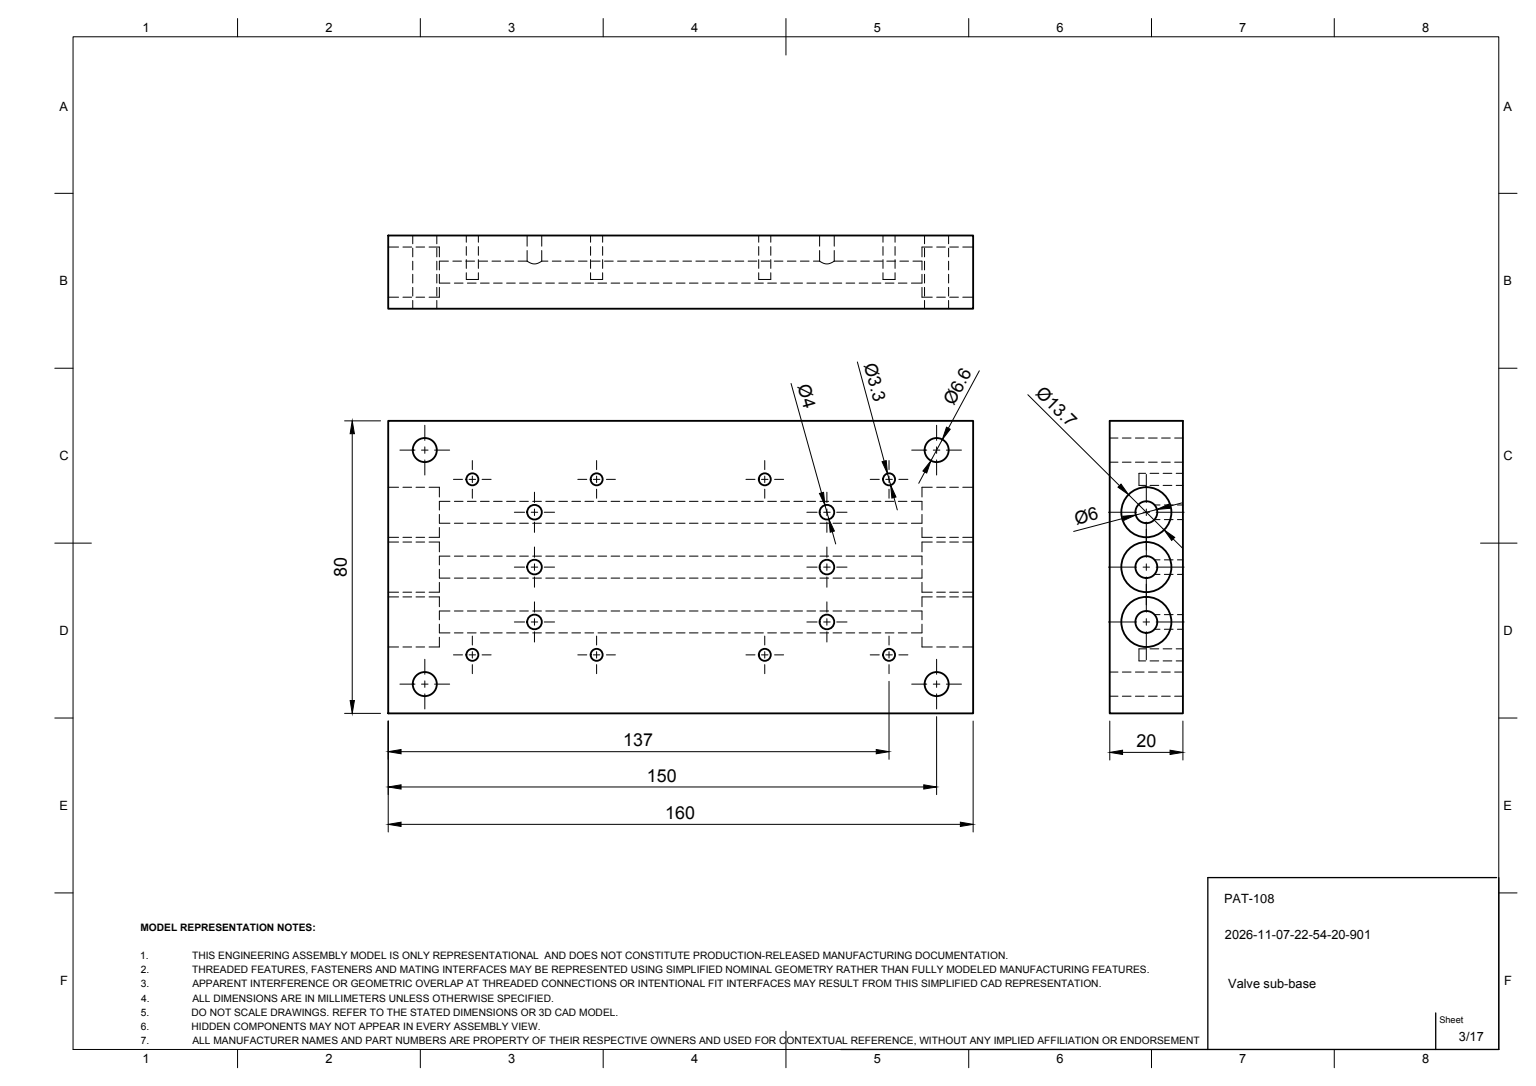
ISO-10303-21;
HEADER;
/* Generated by software containing ST-Developer
 * from STEP Tools, Inc. (www.steptools.com) 
 */

FILE_DESCRIPTION(
/* description */ ('Sub-base valve envelopes and connections'),
/* implementation_level */ '2;1');

FILE_NAME(
/* name */ 'Valve sub-base.step',
/* time_stamp */ '2026-10-29T15:55:44-07:00',
/* author */ (''),
/* organization */ (''),
/* preprocessor_version */ 'ST-DEVELOPER v20.2',
/* originating_system */ 'Autodesk Translation Framework v15.17.0.0',
/* authorisation */ '');

FILE_SCHEMA (('AUTOMOTIVE_DESIGN { 1 0 10303 214 3 1 1 }'));
ENDSEC;

DATA;
#10=MECHANICAL_DESIGN_GEOMETRIC_PRESENTATION_REPRESENTATION('',(#119),#6113);
#95=SHAPE_REPRESENTATION_RELATIONSHIP('SRR','None',#6168,#107);
#107=ADVANCED_BREP_SHAPE_REPRESENTATION('',(#131),#6099);
#119=STYLED_ITEM('',(#6294),#131);
#131=MANIFOLD_SOLID_BREP('Body1',#3358);
#142=FACE_BOUND('',#613,.T.);
#143=FACE_BOUND('',#616,.T.);
#144=FACE_BOUND('',#619,.T.);
#145=FACE_BOUND('',#622,.T.);
#146=FACE_BOUND('',#625,.T.);
#147=FACE_BOUND('',#628,.T.);
#148=FACE_BOUND('',#634,.T.);
#149=FACE_BOUND('',#635,.T.);
#150=FACE_BOUND('',#636,.T.);
#151=FACE_BOUND('',#639,.T.);
#152=FACE_BOUND('',#640,.T.);
#153=FACE_BOUND('',#641,.T.);
#154=FACE_BOUND('',#643,.T.);
#155=FACE_BOUND('',#644,.T.);
#156=FACE_BOUND('',#645,.T.);
#157=FACE_BOUND('',#646,.T.);
#158=FACE_BOUND('',#647,.T.);
#159=FACE_BOUND('',#648,.T.);
#160=FACE_BOUND('',#649,.T.);
#161=FACE_BOUND('',#650,.T.);
#162=FACE_BOUND('',#651,.T.);
#163=FACE_BOUND('',#652,.T.);
#164=FACE_BOUND('',#653,.T.);
#165=FACE_BOUND('',#654,.T.);
#166=FACE_BOUND('',#655,.T.);
#167=FACE_BOUND('',#656,.T.);
#168=FACE_BOUND('',#657,.T.);
#169=FACE_BOUND('',#658,.T.);
#170=FACE_BOUND('',#659,.T.);
#171=FACE_BOUND('',#660,.T.);
#172=FACE_BOUND('',#662,.T.);
#173=FACE_BOUND('',#663,.T.);
#174=FACE_BOUND('',#664,.T.);
#175=FACE_BOUND('',#665,.T.);
#259=B_SPLINE_CURVE_WITH_KNOTS('',3,(#4974,#4975,#4976,#4977,#4978,#4979,
#4980,#4981,#4982,#4983),.UNSPECIFIED.,.F.,.F.,(4,2,2,2,4),(0.,0.0789054703932594,
0.157810940786519,0.235848341776527,0.313885742766534),.UNSPECIFIED.);
#260=B_SPLINE_CURVE_WITH_KNOTS('',3,(#4985,#4986,#4987,#4988,#4989,#4990,
#4991,#4992,#4993,#4994),.UNSPECIFIED.,.F.,.F.,(4,2,2,2,4),(0.941657228299604,
1.01969462928961,1.09773203027962,1.17663750067288,1.25554297106614),
 .UNSPECIFIED.);
#261=B_SPLINE_CURVE_WITH_KNOTS('',3,(#4998,#4999,#5000,#5001,#5002,#5003,
#5004,#5005,#5006,#5007,#5008,#5009,#5010,#5011,#5012,#5013,#5014,#5015),
 .UNSPECIFIED.,.F.,.F.,(4,2,2,2,2,2,2,2,4),(0.313885742766534,0.391923143756543,
0.469960544746551,0.54886601513981,0.627771485533069,0.706676955926329,
0.785582426319588,0.863619827309596,0.941657228299604),.UNSPECIFIED.);
#262=B_SPLINE_CURVE_WITH_KNOTS('',3,(#5019,#5020,#5021,#5022,#5023,#5024,
#5025,#5026,#5027,#5028),.UNSPECIFIED.,.F.,.F.,(4,2,2,2,4),(0.,0.0789054703932594,
0.157810940786519,0.235848341776527,0.313885742766535),.UNSPECIFIED.);
#263=B_SPLINE_CURVE_WITH_KNOTS('',3,(#5030,#5031,#5032,#5033,#5034,#5035,
#5036,#5037,#5038,#5039),.UNSPECIFIED.,.F.,.F.,(4,2,2,2,4),(0.941657228299605,
1.01969462928961,1.09773203027962,1.17663750067288,1.25554297106614),
 .UNSPECIFIED.);
#264=B_SPLINE_CURVE_WITH_KNOTS('',3,(#5043,#5044,#5045,#5046,#5047,#5048,
#5049,#5050,#5051,#5052,#5053,#5054,#5055,#5056,#5057,#5058,#5059,#5060),
 .UNSPECIFIED.,.F.,.F.,(4,2,2,2,2,2,2,2,4),(0.313885742766535,0.391923143756543,
0.469960544746551,0.54886601513981,0.627771485533069,0.706676955926329,
0.785582426319588,0.863619827309597,0.941657228299605),.UNSPECIFIED.);
#265=B_SPLINE_CURVE_WITH_KNOTS('',3,(#5064,#5065,#5066,#5067,#5068,#5069,
#5070,#5071,#5072,#5073),.UNSPECIFIED.,.F.,.F.,(4,2,2,2,4),(0.,0.0789054703932594,
0.157810940786519,0.235848341776527,0.313885742766534),.UNSPECIFIED.);
#266=B_SPLINE_CURVE_WITH_KNOTS('',3,(#5075,#5076,#5077,#5078,#5079,#5080,
#5081,#5082,#5083,#5084),.UNSPECIFIED.,.F.,.F.,(4,2,2,2,4),(0.941657228299604,
1.01969462928961,1.09773203027962,1.17663750067288,1.25554297106614),
 .UNSPECIFIED.);
#267=B_SPLINE_CURVE_WITH_KNOTS('',3,(#5088,#5089,#5090,#5091,#5092,#5093,
#5094,#5095,#5096,#5097,#5098,#5099,#5100,#5101,#5102,#5103,#5104,#5105),
 .UNSPECIFIED.,.F.,.F.,(4,2,2,2,2,2,2,2,4),(0.313885742766534,0.391923143756543,
0.469960544746551,0.54886601513981,0.627771485533069,0.706676955926329,
0.785582426319588,0.863619827309596,0.941657228299604),.UNSPECIFIED.);
#268=B_SPLINE_CURVE_WITH_KNOTS('',3,(#5137,#5138,#5139,#5140,#5141,#5142,
#5143,#5144,#5145,#5146),.UNSPECIFIED.,.F.,.F.,(4,2,2,2,4),(0.,0.0789054703932594,
0.157810940786519,0.235848341776527,0.313885742766535),.UNSPECIFIED.);
#269=B_SPLINE_CURVE_WITH_KNOTS('',3,(#5148,#5149,#5150,#5151,#5152,#5153,
#5154,#5155,#5156,#5157),.UNSPECIFIED.,.F.,.F.,(4,2,2,2,4),(0.941657228299605,
1.01969462928961,1.09773203027962,1.17663750067288,1.25554297106614),
 .UNSPECIFIED.);
#270=B_SPLINE_CURVE_WITH_KNOTS('',3,(#5161,#5162,#5163,#5164,#5165,#5166,
#5167,#5168,#5169,#5170,#5171,#5172,#5173,#5174,#5175,#5176,#5177,#5178),
 .UNSPECIFIED.,.F.,.F.,(4,2,2,2,2,2,2,2,4),(0.313885742766535,0.391923143756543,
0.469960544746551,0.54886601513981,0.62777148553307,0.706676955926329,0.785582426319589,
0.863619827309597,0.941657228299605),.UNSPECIFIED.);
#271=B_SPLINE_CURVE_WITH_KNOTS('',3,(#5182,#5183,#5184,#5185,#5186,#5187,
#5188,#5189,#5190,#5191),.UNSPECIFIED.,.F.,.F.,(4,2,2,2,4),(0.,0.0789054703932594,
0.157810940786519,0.235848341776527,0.313885742766535),.UNSPECIFIED.);
#272=B_SPLINE_CURVE_WITH_KNOTS('',3,(#5193,#5194,#5195,#5196,#5197,#5198,
#5199,#5200,#5201,#5202),.UNSPECIFIED.,.F.,.F.,(4,2,2,2,4),(0.941657228299605,
1.01969462928961,1.09773203027962,1.17663750067288,1.25554297106614),
 .UNSPECIFIED.);
#273=B_SPLINE_CURVE_WITH_KNOTS('',3,(#5206,#5207,#5208,#5209,#5210,#5211,
#5212,#5213,#5214,#5215,#5216,#5217,#5218,#5219,#5220,#5221,#5222,#5223),
 .UNSPECIFIED.,.F.,.F.,(4,2,2,2,2,2,2,2,4),(0.313885742766535,0.391923143756543,
0.469960544746551,0.548866015139811,0.62777148553307,0.706676955926329,
0.785582426319589,0.863619827309597,0.941657228299605),.UNSPECIFIED.);
#274=B_SPLINE_CURVE_WITH_KNOTS('',3,(#5227,#5228,#5229,#5230,#5231,#5232,
#5233,#5234,#5235,#5236),.UNSPECIFIED.,.F.,.F.,(4,2,2,2,4),(0.,0.0789054703932594,
0.157810940786519,0.235848341776527,0.313885742766535),.UNSPECIFIED.);
#275=B_SPLINE_CURVE_WITH_KNOTS('',3,(#5238,#5239,#5240,#5241,#5242,#5243,
#5244,#5245,#5246,#5247),.UNSPECIFIED.,.F.,.F.,(4,2,2,2,4),(0.941657228299605,
1.01969462928961,1.09773203027962,1.17663750067288,1.25554297106614),
 .UNSPECIFIED.);
#276=B_SPLINE_CURVE_WITH_KNOTS('',3,(#5251,#5252,#5253,#5254,#5255,#5256,
#5257,#5258,#5259,#5260,#5261,#5262,#5263,#5264,#5265,#5266,#5267,#5268),
 .UNSPECIFIED.,.F.,.F.,(4,2,2,2,2,2,2,2,4),(0.313885742766535,0.391923143756543,
0.469960544746551,0.54886601513981,0.62777148553307,0.706676955926329,0.785582426319589,
0.863619827309597,0.941657228299605),.UNSPECIFIED.);
#277=PLANE('',#3509);
#278=PLANE('',#3513);
#279=PLANE('',#3517);
#280=PLANE('',#3521);
#281=PLANE('',#3531);
#282=PLANE('',#3535);
#283=PLANE('',#3539);
#284=PLANE('',#3543);
#285=PLANE('',#3565);
#286=PLANE('',#3570);
#287=PLANE('',#3575);
#288=PLANE('',#3580);
#289=PLANE('',#3585);
#290=PLANE('',#3590);
#291=PLANE('',#3595);
#292=PLANE('',#3596);
#293=PLANE('',#3597);
#294=PLANE('',#3598);
#295=PLANE('',#3599);
#296=PLANE('',#3600);
#386=FACE_OUTER_BOUND('',#585,.T.);
#387=FACE_OUTER_BOUND('',#586,.T.);
#388=FACE_OUTER_BOUND('',#587,.T.);
#389=FACE_OUTER_BOUND('',#588,.T.);
#390=FACE_OUTER_BOUND('',#589,.T.);
#391=FACE_OUTER_BOUND('',#590,.T.);
#392=FACE_OUTER_BOUND('',#591,.T.);
#393=FACE_OUTER_BOUND('',#592,.T.);
#394=FACE_OUTER_BOUND('',#593,.T.);
#395=FACE_OUTER_BOUND('',#594,.T.);
#396=FACE_OUTER_BOUND('',#595,.T.);
#397=FACE_OUTER_BOUND('',#596,.T.);
#398=FACE_OUTER_BOUND('',#597,.T.);
#399=FACE_OUTER_BOUND('',#598,.T.);
#400=FACE_OUTER_BOUND('',#599,.T.);
#401=FACE_OUTER_BOUND('',#600,.T.);
#402=FACE_OUTER_BOUND('',#601,.T.);
#403=FACE_OUTER_BOUND('',#602,.T.);
#404=FACE_OUTER_BOUND('',#603,.T.);
#405=FACE_OUTER_BOUND('',#604,.T.);
#406=FACE_OUTER_BOUND('',#605,.T.);
#407=FACE_OUTER_BOUND('',#606,.T.);
#408=FACE_OUTER_BOUND('',#607,.T.);
#409=FACE_OUTER_BOUND('',#608,.T.);
#410=FACE_OUTER_BOUND('',#609,.T.);
#411=FACE_OUTER_BOUND('',#610,.T.);
#412=FACE_OUTER_BOUND('',#611,.T.);
#413=FACE_OUTER_BOUND('',#612,.T.);
#414=FACE_OUTER_BOUND('',#614,.T.);
#415=FACE_OUTER_BOUND('',#615,.T.);
#416=FACE_OUTER_BOUND('',#617,.T.);
#417=FACE_OUTER_BOUND('',#618,.T.);
#418=FACE_OUTER_BOUND('',#620,.T.);
#419=FACE_OUTER_BOUND('',#621,.T.);
#420=FACE_OUTER_BOUND('',#623,.T.);
#421=FACE_OUTER_BOUND('',#624,.T.);
#422=FACE_OUTER_BOUND('',#626,.T.);
#423=FACE_OUTER_BOUND('',#627,.T.);
#424=FACE_OUTER_BOUND('',#629,.T.);
#425=FACE_OUTER_BOUND('',#630,.T.);
#426=FACE_OUTER_BOUND('',#631,.T.);
#427=FACE_OUTER_BOUND('',#632,.T.);
#428=FACE_OUTER_BOUND('',#633,.T.);
#429=FACE_OUTER_BOUND('',#637,.T.);
#430=FACE_OUTER_BOUND('',#638,.T.);
#431=FACE_OUTER_BOUND('',#642,.T.);
#432=FACE_OUTER_BOUND('',#661,.T.);
#585=EDGE_LOOP('',(#2235,#2236,#2237,#2238));
#586=EDGE_LOOP('',(#2239));
#587=EDGE_LOOP('',(#2240,#2241,#2242,#2243));
#588=EDGE_LOOP('',(#2244));
#589=EDGE_LOOP('',(#2245,#2246,#2247,#2248));
#590=EDGE_LOOP('',(#2249));
#591=EDGE_LOOP('',(#2250,#2251,#2252,#2253));
#592=EDGE_LOOP('',(#2254));
#593=EDGE_LOOP('',(#2255,#2256,#2257,#2258,#2259,#2260));
#594=EDGE_LOOP('',(#2261,#2262,#2263,#2264,#2265,#2266));
#595=EDGE_LOOP('',(#2267,#2268,#2269,#2270,#2271,#2272));
#596=EDGE_LOOP('',(#2273,#2274,#2275,#2276));
#597=EDGE_LOOP('',(#2277));
#598=EDGE_LOOP('',(#2278,#2279,#2280,#2281));
#599=EDGE_LOOP('',(#2282));
#600=EDGE_LOOP('',(#2283,#2284,#2285,#2286));
#601=EDGE_LOOP('',(#2287));
#602=EDGE_LOOP('',(#2288,#2289,#2290,#2291));
#603=EDGE_LOOP('',(#2292));
#604=EDGE_LOOP('',(#2293,#2294,#2295,#2296,#2297,#2298));
#605=EDGE_LOOP('',(#2299,#2300,#2301,#2302,#2303,#2304));
#606=EDGE_LOOP('',(#2305,#2306,#2307,#2308,#2309,#2310));
#607=EDGE_LOOP('',(#2311,#2312,#2313,#2314));
#608=EDGE_LOOP('',(#2315,#2316,#2317,#2318));
#609=EDGE_LOOP('',(#2319,#2320,#2321,#2322));
#610=EDGE_LOOP('',(#2323,#2324,#2325,#2326));
#611=EDGE_LOOP('',(#2327,#2328,#2329,#2330));
#612=EDGE_LOOP('',(#2331));
#613=EDGE_LOOP('',(#2332));
#614=EDGE_LOOP('',(#2333,#2334,#2335,#2336));
#615=EDGE_LOOP('',(#2337));
#616=EDGE_LOOP('',(#2338));
#617=EDGE_LOOP('',(#2339,#2340,#2341,#2342));
#618=EDGE_LOOP('',(#2343));
#619=EDGE_LOOP('',(#2344));
#620=EDGE_LOOP('',(#2345,#2346,#2347,#2348));
#621=EDGE_LOOP('',(#2349));
#622=EDGE_LOOP('',(#2350));
#623=EDGE_LOOP('',(#2351,#2352,#2353,#2354));
#624=EDGE_LOOP('',(#2355));
#625=EDGE_LOOP('',(#2356));
#626=EDGE_LOOP('',(#2357,#2358,#2359,#2360));
#627=EDGE_LOOP('',(#2361));
#628=EDGE_LOOP('',(#2362));
#629=EDGE_LOOP('',(#2363,#2364,#2365,#2366,#2367,#2368,#2369,#2370,#2371,
#2372,#2373,#2374,#2375,#2376));
#630=EDGE_LOOP('',(#2377,#2378,#2379,#2380,#2381,#2382,#2383,#2384,#2385,
#2386,#2387,#2388,#2389,#2390));
#631=EDGE_LOOP('',(#2391,#2392,#2393,#2394,#2395,#2396,#2397,#2398,#2399,
#2400,#2401,#2402,#2403,#2404));
#632=EDGE_LOOP('',(#2405,#2406,#2407,#2408));
#633=EDGE_LOOP('',(#2409,#2410,#2411,#2412));
#634=EDGE_LOOP('',(#2413));
#635=EDGE_LOOP('',(#2414));
#636=EDGE_LOOP('',(#2415));
#637=EDGE_LOOP('',(#2416,#2417,#2418,#2419));
#638=EDGE_LOOP('',(#2420,#2421,#2422,#2423));
#639=EDGE_LOOP('',(#2424));
#640=EDGE_LOOP('',(#2425));
#641=EDGE_LOOP('',(#2426));
#642=EDGE_LOOP('',(#2427,#2428,#2429,#2430));
#643=EDGE_LOOP('',(#2431));
#644=EDGE_LOOP('',(#2432));
#645=EDGE_LOOP('',(#2433));
#646=EDGE_LOOP('',(#2434));
#647=EDGE_LOOP('',(#2435));
#648=EDGE_LOOP('',(#2436));
#649=EDGE_LOOP('',(#2437));
#650=EDGE_LOOP('',(#2438));
#651=EDGE_LOOP('',(#2439));
#652=EDGE_LOOP('',(#2440));
#653=EDGE_LOOP('',(#2441));
#654=EDGE_LOOP('',(#2442));
#655=EDGE_LOOP('',(#2443));
#656=EDGE_LOOP('',(#2444));
#657=EDGE_LOOP('',(#2445));
#658=EDGE_LOOP('',(#2446));
#659=EDGE_LOOP('',(#2447));
#660=EDGE_LOOP('',(#2448));
#661=EDGE_LOOP('',(#2449,#2450,#2451,#2452));
#662=EDGE_LOOP('',(#2453));
#663=EDGE_LOOP('',(#2454));
#664=EDGE_LOOP('',(#2455));
#665=EDGE_LOOP('',(#2456));
#901=LINE('',#4947,#1135);
#902=LINE('',#4954,#1136);
#903=LINE('',#4961,#1137);
#904=LINE('',#4968,#1138);
#905=LINE('',#4996,#1139);
#906=LINE('',#5041,#1140);
#907=LINE('',#5086,#1141);
#908=LINE('',#5110,#1142);
#909=LINE('',#5117,#1143);
#910=LINE('',#5124,#1144);
#911=LINE('',#5131,#1145);
#912=LINE('',#5159,#1146);
#913=LINE('',#5204,#1147);
#914=LINE('',#5249,#1148);
#915=LINE('',#5273,#1149);
#916=LINE('',#5279,#1150);
#917=LINE('',#5285,#1151);
#918=LINE('',#5291,#1152);
#919=LINE('',#5297,#1153);
#920=LINE('',#5306,#1154);
#921=LINE('',#5315,#1155);
#922=LINE('',#5324,#1156);
#923=LINE('',#5333,#1157);
#924=LINE('',#5342,#1158);
#925=LINE('',#5348,#1159);
#926=LINE('',#5349,#1160);
#927=LINE('',#5350,#1161);
#928=LINE('',#5352,#1162);
#929=LINE('',#5353,#1163);
#930=LINE('',#5354,#1164);
#931=LINE('',#5356,#1165);
#932=LINE('',#5357,#1166);
#933=LINE('',#5358,#1167);
#934=LINE('',#5362,#1168);
#935=LINE('',#5364,#1169);
#936=LINE('',#5366,#1170);
#937=LINE('',#5367,#1171);
#938=LINE('',#5370,#1172);
#939=LINE('',#5372,#1173);
#940=LINE('',#5373,#1174);
#941=LINE('',#5376,#1175);
#942=LINE('',#5378,#1176);
#943=LINE('',#5379,#1177);
#944=LINE('',#5381,#1178);
#945=LINE('',#5382,#1179);
#1135=VECTOR('',#3913,0.165);
#1136=VECTOR('',#3922,0.165);
#1137=VECTOR('',#3931,0.165);
#1138=VECTOR('',#3940,0.165);
#1139=VECTOR('',#3947,0.2);
#1140=VECTOR('',#3952,0.2);
#1141=VECTOR('',#3957,0.2);
#1142=VECTOR('',#3964,0.165);
#1143=VECTOR('',#3973,0.165);
#1144=VECTOR('',#3982,0.165);
#1145=VECTOR('',#3991,0.165);
#1146=VECTOR('',#3998,0.2);
#1147=VECTOR('',#4003,0.2);
#1148=VECTOR('',#4008,0.2);
#1149=VECTOR('',#4015,0.33);
#1150=VECTOR('',#4022,0.33);
#1151=VECTOR('',#4029,0.33);
#1152=VECTOR('',#4036,0.33);
#1153=VECTOR('',#4043,0.685);
#1154=VECTOR('',#4054,0.685);
#1155=VECTOR('',#4065,0.685);
#1156=VECTOR('',#4076,0.685);
#1157=VECTOR('',#4087,0.685);
#1158=VECTOR('',#4098,0.685);
#1159=VECTOR('',#4107,0.3);
#1160=VECTOR('',#4108,0.3);
#1161=VECTOR('',#4109,0.3);
#1162=VECTOR('',#4112,0.3);
#1163=VECTOR('',#4113,0.3);
#1164=VECTOR('',#4114,0.3);
#1165=VECTOR('',#4117,0.3);
#1166=VECTOR('',#4118,0.3);
#1167=VECTOR('',#4119,0.3);
#1168=VECTOR('',#4122,1.);
#1169=VECTOR('',#4123,1.);
#1170=VECTOR('',#4124,1.);
#1171=VECTOR('',#4125,1.);
#1172=VECTOR('',#4128,1.);
#1173=VECTOR('',#4129,1.);
#1174=VECTOR('',#4130,1.);
#1175=VECTOR('',#4133,1.);
#1176=VECTOR('',#4134,1.);
#1177=VECTOR('',#4135,1.);
#1178=VECTOR('',#4138,1.);
#1179=VECTOR('',#4139,1.);
#1369=CIRCLE('',#3507,0.165);
#1370=CIRCLE('',#3508,0.165);
#1371=CIRCLE('',#3511,0.165);
#1372=CIRCLE('',#3512,0.165);
#1373=CIRCLE('',#3515,0.165);
#1374=CIRCLE('',#3516,0.165);
#1375=CIRCLE('',#3519,0.165);
#1376=CIRCLE('',#3520,0.165);
#1377=CIRCLE('',#3523,0.2);
#1378=CIRCLE('',#3525,0.2);
#1379=CIRCLE('',#3527,0.2);
#1380=CIRCLE('',#3529,0.165);
#1381=CIRCLE('',#3530,0.165);
#1382=CIRCLE('',#3533,0.165);
#1383=CIRCLE('',#3534,0.165);
#1384=CIRCLE('',#3537,0.165);
#1385=CIRCLE('',#3538,0.165);
#1386=CIRCLE('',#3541,0.165);
#1387=CIRCLE('',#3542,0.165);
#1388=CIRCLE('',#3545,0.2);
#1389=CIRCLE('',#3547,0.2);
#1390=CIRCLE('',#3549,0.2);
#1391=CIRCLE('',#3551,0.33);
#1392=CIRCLE('',#3552,0.33);
#1393=CIRCLE('',#3554,0.33);
#1394=CIRCLE('',#3555,0.33);
#1395=CIRCLE('',#3557,0.33);
#1396=CIRCLE('',#3558,0.33);
#1397=CIRCLE('',#3560,0.33);
#1398=CIRCLE('',#3561,0.33);
#1399=CIRCLE('',#3563,0.685);
#1400=CIRCLE('',#3564,0.685);
#1401=CIRCLE('',#3566,0.3);
#1402=CIRCLE('',#3568,0.685);
#1403=CIRCLE('',#3569,0.685);
#1404=CIRCLE('',#3571,0.3);
#1405=CIRCLE('',#3573,0.685);
#1406=CIRCLE('',#3574,0.685);
#1407=CIRCLE('',#3576,0.3);
#1408=CIRCLE('',#3578,0.685);
#1409=CIRCLE('',#3579,0.685);
#1410=CIRCLE('',#3581,0.3);
#1411=CIRCLE('',#3583,0.685);
#1412=CIRCLE('',#3584,0.685);
#1413=CIRCLE('',#3586,0.3);
#1414=CIRCLE('',#3588,0.685);
#1415=CIRCLE('',#3589,0.685);
#1416=CIRCLE('',#3591,0.3);
#1537=VERTEX_POINT('',#4944);
#1538=VERTEX_POINT('',#4946);
#1539=VERTEX_POINT('',#4951);
#1540=VERTEX_POINT('',#4953);
#1541=VERTEX_POINT('',#4958);
#1542=VERTEX_POINT('',#4960);
#1543=VERTEX_POINT('',#4965);
#1544=VERTEX_POINT('',#4967);
#1545=VERTEX_POINT('',#4972);
#1546=VERTEX_POINT('',#4973);
#1547=VERTEX_POINT('',#4984);
#1548=VERTEX_POINT('',#4995);
#1549=VERTEX_POINT('',#5017);
#1550=VERTEX_POINT('',#5018);
#1551=VERTEX_POINT('',#5029);
#1552=VERTEX_POINT('',#5040);
#1553=VERTEX_POINT('',#5062);
#1554=VERTEX_POINT('',#5063);
#1555=VERTEX_POINT('',#5074);
#1556=VERTEX_POINT('',#5085);
#1557=VERTEX_POINT('',#5107);
#1558=VERTEX_POINT('',#5109);
#1559=VERTEX_POINT('',#5114);
#1560=VERTEX_POINT('',#5116);
#1561=VERTEX_POINT('',#5121);
#1562=VERTEX_POINT('',#5123);
#1563=VERTEX_POINT('',#5128);
#1564=VERTEX_POINT('',#5130);
#1565=VERTEX_POINT('',#5135);
#1566=VERTEX_POINT('',#5136);
#1567=VERTEX_POINT('',#5147);
#1568=VERTEX_POINT('',#5158);
#1569=VERTEX_POINT('',#5180);
#1570=VERTEX_POINT('',#5181);
#1571=VERTEX_POINT('',#5192);
#1572=VERTEX_POINT('',#5203);
#1573=VERTEX_POINT('',#5225);
#1574=VERTEX_POINT('',#5226);
#1575=VERTEX_POINT('',#5237);
#1576=VERTEX_POINT('',#5248);
#1577=VERTEX_POINT('',#5270);
#1578=VERTEX_POINT('',#5272);
#1579=VERTEX_POINT('',#5276);
#1580=VERTEX_POINT('',#5278);
#1581=VERTEX_POINT('',#5282);
#1582=VERTEX_POINT('',#5284);
#1583=VERTEX_POINT('',#5288);
#1584=VERTEX_POINT('',#5290);
#1585=VERTEX_POINT('',#5294);
#1586=VERTEX_POINT('',#5296);
#1587=VERTEX_POINT('',#5300);
#1588=VERTEX_POINT('',#5303);
#1589=VERTEX_POINT('',#5305);
#1590=VERTEX_POINT('',#5309);
#1591=VERTEX_POINT('',#5312);
#1592=VERTEX_POINT('',#5314);
#1593=VERTEX_POINT('',#5318);
#1594=VERTEX_POINT('',#5321);
#1595=VERTEX_POINT('',#5323);
#1596=VERTEX_POINT('',#5327);
#1597=VERTEX_POINT('',#5330);
#1598=VERTEX_POINT('',#5332);
#1599=VERTEX_POINT('',#5336);
#1600=VERTEX_POINT('',#5339);
#1601=VERTEX_POINT('',#5341);
#1602=VERTEX_POINT('',#5345);
#1603=VERTEX_POINT('',#5360);
#1604=VERTEX_POINT('',#5361);
#1605=VERTEX_POINT('',#5363);
#1606=VERTEX_POINT('',#5365);
#1607=VERTEX_POINT('',#5369);
#1608=VERTEX_POINT('',#5371);
#1609=VERTEX_POINT('',#5375);
#1610=VERTEX_POINT('',#5377);
#1815=EDGE_CURVE('',#1537,#1537,#1369,.T.);
#1816=EDGE_CURVE('',#1537,#1538,#901,.T.);
#1817=EDGE_CURVE('',#1538,#1538,#1370,.T.);
#1818=EDGE_CURVE('',#1539,#1539,#1371,.T.);
#1819=EDGE_CURVE('',#1539,#1540,#902,.T.);
#1820=EDGE_CURVE('',#1540,#1540,#1372,.T.);
#1821=EDGE_CURVE('',#1541,#1541,#1373,.T.);
#1822=EDGE_CURVE('',#1541,#1542,#903,.T.);
#1823=EDGE_CURVE('',#1542,#1542,#1374,.T.);
#1824=EDGE_CURVE('',#1543,#1543,#1375,.T.);
#1825=EDGE_CURVE('',#1543,#1544,#904,.T.);
#1826=EDGE_CURVE('',#1544,#1544,#1376,.T.);
#1827=EDGE_CURVE('',#1545,#1546,#259,.T.);
#1828=EDGE_CURVE('',#1547,#1545,#260,.T.);
#1829=EDGE_CURVE('',#1547,#1548,#905,.T.);
#1830=EDGE_CURVE('',#1548,#1548,#1377,.T.);
#1831=EDGE_CURVE('',#1546,#1547,#261,.T.);
#1832=EDGE_CURVE('',#1549,#1550,#262,.T.);
#1833=EDGE_CURVE('',#1551,#1549,#263,.T.);
#1834=EDGE_CURVE('',#1551,#1552,#906,.T.);
#1835=EDGE_CURVE('',#1552,#1552,#1378,.T.);
#1836=EDGE_CURVE('',#1550,#1551,#264,.T.);
#1837=EDGE_CURVE('',#1553,#1554,#265,.T.);
#1838=EDGE_CURVE('',#1555,#1553,#266,.T.);
#1839=EDGE_CURVE('',#1555,#1556,#907,.T.);
#1840=EDGE_CURVE('',#1556,#1556,#1379,.T.);
#1841=EDGE_CURVE('',#1554,#1555,#267,.T.);
#1842=EDGE_CURVE('',#1557,#1557,#1380,.T.);
#1843=EDGE_CURVE('',#1557,#1558,#908,.T.);
#1844=EDGE_CURVE('',#1558,#1558,#1381,.T.);
#1845=EDGE_CURVE('',#1559,#1559,#1382,.T.);
#1846=EDGE_CURVE('',#1559,#1560,#909,.T.);
#1847=EDGE_CURVE('',#1560,#1560,#1383,.T.);
#1848=EDGE_CURVE('',#1561,#1561,#1384,.T.);
#1849=EDGE_CURVE('',#1561,#1562,#910,.T.);
#1850=EDGE_CURVE('',#1562,#1562,#1385,.T.);
#1851=EDGE_CURVE('',#1563,#1563,#1386,.T.);
#1852=EDGE_CURVE('',#1563,#1564,#911,.T.);
#1853=EDGE_CURVE('',#1564,#1564,#1387,.T.);
#1854=EDGE_CURVE('',#1565,#1566,#268,.T.);
#1855=EDGE_CURVE('',#1567,#1565,#269,.T.);
#1856=EDGE_CURVE('',#1567,#1568,#912,.T.);
#1857=EDGE_CURVE('',#1568,#1568,#1388,.T.);
#1858=EDGE_CURVE('',#1566,#1567,#270,.T.);
#1859=EDGE_CURVE('',#1569,#1570,#271,.T.);
#1860=EDGE_CURVE('',#1571,#1569,#272,.T.);
#1861=EDGE_CURVE('',#1571,#1572,#913,.T.);
#1862=EDGE_CURVE('',#1572,#1572,#1389,.T.);
#1863=EDGE_CURVE('',#1570,#1571,#273,.T.);
#1864=EDGE_CURVE('',#1573,#1574,#274,.T.);
#1865=EDGE_CURVE('',#1575,#1573,#275,.T.);
#1866=EDGE_CURVE('',#1575,#1576,#914,.T.);
#1867=EDGE_CURVE('',#1576,#1576,#1390,.T.);
#1868=EDGE_CURVE('',#1574,#1575,#276,.T.);
#1869=EDGE_CURVE('',#1577,#1577,#1391,.T.);
#1870=EDGE_CURVE('',#1577,#1578,#915,.T.);
#1871=EDGE_CURVE('',#1578,#1578,#1392,.T.);
#1872=EDGE_CURVE('',#1579,#1579,#1393,.T.);
#1873=EDGE_CURVE('',#1579,#1580,#916,.T.);
#1874=EDGE_CURVE('',#1580,#1580,#1394,.T.);
#1875=EDGE_CURVE('',#1581,#1581,#1395,.T.);
#1876=EDGE_CURVE('',#1581,#1582,#917,.T.);
#1877=EDGE_CURVE('',#1582,#1582,#1396,.T.);
#1878=EDGE_CURVE('',#1583,#1583,#1397,.T.);
#1879=EDGE_CURVE('',#1583,#1584,#918,.T.);
#1880=EDGE_CURVE('',#1584,#1584,#1398,.T.);
#1881=EDGE_CURVE('',#1585,#1585,#1399,.T.);
#1882=EDGE_CURVE('',#1585,#1586,#919,.T.);
#1883=EDGE_CURVE('',#1586,#1586,#1400,.T.);
#1884=EDGE_CURVE('',#1587,#1587,#1401,.T.);
#1885=EDGE_CURVE('',#1588,#1588,#1402,.T.);
#1886=EDGE_CURVE('',#1588,#1589,#920,.T.);
#1887=EDGE_CURVE('',#1589,#1589,#1403,.T.);
#1888=EDGE_CURVE('',#1590,#1590,#1404,.T.);
#1889=EDGE_CURVE('',#1591,#1591,#1405,.T.);
#1890=EDGE_CURVE('',#1591,#1592,#921,.T.);
#1891=EDGE_CURVE('',#1592,#1592,#1406,.T.);
#1892=EDGE_CURVE('',#1593,#1593,#1407,.T.);
#1893=EDGE_CURVE('',#1594,#1594,#1408,.T.);
#1894=EDGE_CURVE('',#1594,#1595,#922,.T.);
#1895=EDGE_CURVE('',#1595,#1595,#1409,.T.);
#1896=EDGE_CURVE('',#1596,#1596,#1410,.T.);
#1897=EDGE_CURVE('',#1597,#1597,#1411,.T.);
#1898=EDGE_CURVE('',#1597,#1598,#923,.T.);
#1899=EDGE_CURVE('',#1598,#1598,#1412,.T.);
#1900=EDGE_CURVE('',#1599,#1599,#1413,.T.);
#1901=EDGE_CURVE('',#1600,#1600,#1414,.T.);
#1902=EDGE_CURVE('',#1600,#1601,#924,.T.);
#1903=EDGE_CURVE('',#1601,#1601,#1415,.T.);
#1904=EDGE_CURVE('',#1602,#1602,#1416,.T.);
#1905=EDGE_CURVE('',#1596,#1567,#925,.T.);
#1906=EDGE_CURVE('',#1566,#1547,#926,.T.);
#1907=EDGE_CURVE('',#1546,#1587,#927,.T.);
#1908=EDGE_CURVE('',#1599,#1571,#928,.T.);
#1909=EDGE_CURVE('',#1570,#1551,#929,.T.);
#1910=EDGE_CURVE('',#1550,#1590,#930,.T.);
#1911=EDGE_CURVE('',#1602,#1575,#931,.T.);
#1912=EDGE_CURVE('',#1574,#1555,#932,.T.);
#1913=EDGE_CURVE('',#1554,#1593,#933,.T.);
#1914=EDGE_CURVE('',#1603,#1604,#934,.T.);
#1915=EDGE_CURVE('',#1604,#1605,#935,.T.);
#1916=EDGE_CURVE('',#1606,#1605,#936,.T.);
#1917=EDGE_CURVE('',#1603,#1606,#937,.T.);
#1918=EDGE_CURVE('',#1607,#1603,#938,.T.);
#1919=EDGE_CURVE('',#1608,#1606,#939,.T.);
#1920=EDGE_CURVE('',#1607,#1608,#940,.T.);
#1921=EDGE_CURVE('',#1609,#1607,#941,.T.);
#1922=EDGE_CURVE('',#1610,#1608,#942,.T.);
#1923=EDGE_CURVE('',#1609,#1610,#943,.T.);
#1924=EDGE_CURVE('',#1604,#1609,#944,.T.);
#1925=EDGE_CURVE('',#1605,#1610,#945,.T.);
#2235=ORIENTED_EDGE('',*,*,#1815,.F.);
#2236=ORIENTED_EDGE('',*,*,#1816,.T.);
#2237=ORIENTED_EDGE('',*,*,#1817,.F.);
#2238=ORIENTED_EDGE('',*,*,#1816,.F.);
#2239=ORIENTED_EDGE('',*,*,#1815,.T.);
#2240=ORIENTED_EDGE('',*,*,#1818,.F.);
#2241=ORIENTED_EDGE('',*,*,#1819,.T.);
#2242=ORIENTED_EDGE('',*,*,#1820,.F.);
#2243=ORIENTED_EDGE('',*,*,#1819,.F.);
#2244=ORIENTED_EDGE('',*,*,#1818,.T.);
#2245=ORIENTED_EDGE('',*,*,#1821,.F.);
#2246=ORIENTED_EDGE('',*,*,#1822,.T.);
#2247=ORIENTED_EDGE('',*,*,#1823,.F.);
#2248=ORIENTED_EDGE('',*,*,#1822,.F.);
#2249=ORIENTED_EDGE('',*,*,#1821,.T.);
#2250=ORIENTED_EDGE('',*,*,#1824,.F.);
#2251=ORIENTED_EDGE('',*,*,#1825,.T.);
#2252=ORIENTED_EDGE('',*,*,#1826,.F.);
#2253=ORIENTED_EDGE('',*,*,#1825,.F.);
#2254=ORIENTED_EDGE('',*,*,#1824,.T.);
#2255=ORIENTED_EDGE('',*,*,#1827,.F.);
#2256=ORIENTED_EDGE('',*,*,#1828,.F.);
#2257=ORIENTED_EDGE('',*,*,#1829,.T.);
#2258=ORIENTED_EDGE('',*,*,#1830,.F.);
#2259=ORIENTED_EDGE('',*,*,#1829,.F.);
#2260=ORIENTED_EDGE('',*,*,#1831,.F.);
#2261=ORIENTED_EDGE('',*,*,#1832,.F.);
#2262=ORIENTED_EDGE('',*,*,#1833,.F.);
#2263=ORIENTED_EDGE('',*,*,#1834,.T.);
#2264=ORIENTED_EDGE('',*,*,#1835,.F.);
#2265=ORIENTED_EDGE('',*,*,#1834,.F.);
#2266=ORIENTED_EDGE('',*,*,#1836,.F.);
#2267=ORIENTED_EDGE('',*,*,#1837,.F.);
#2268=ORIENTED_EDGE('',*,*,#1838,.F.);
#2269=ORIENTED_EDGE('',*,*,#1839,.T.);
#2270=ORIENTED_EDGE('',*,*,#1840,.F.);
#2271=ORIENTED_EDGE('',*,*,#1839,.F.);
#2272=ORIENTED_EDGE('',*,*,#1841,.F.);
#2273=ORIENTED_EDGE('',*,*,#1842,.F.);
#2274=ORIENTED_EDGE('',*,*,#1843,.T.);
#2275=ORIENTED_EDGE('',*,*,#1844,.F.);
#2276=ORIENTED_EDGE('',*,*,#1843,.F.);
#2277=ORIENTED_EDGE('',*,*,#1842,.T.);
#2278=ORIENTED_EDGE('',*,*,#1845,.F.);
#2279=ORIENTED_EDGE('',*,*,#1846,.T.);
#2280=ORIENTED_EDGE('',*,*,#1847,.F.);
#2281=ORIENTED_EDGE('',*,*,#1846,.F.);
#2282=ORIENTED_EDGE('',*,*,#1845,.T.);
#2283=ORIENTED_EDGE('',*,*,#1848,.F.);
#2284=ORIENTED_EDGE('',*,*,#1849,.T.);
#2285=ORIENTED_EDGE('',*,*,#1850,.F.);
#2286=ORIENTED_EDGE('',*,*,#1849,.F.);
#2287=ORIENTED_EDGE('',*,*,#1848,.T.);
#2288=ORIENTED_EDGE('',*,*,#1851,.F.);
#2289=ORIENTED_EDGE('',*,*,#1852,.T.);
#2290=ORIENTED_EDGE('',*,*,#1853,.F.);
#2291=ORIENTED_EDGE('',*,*,#1852,.F.);
#2292=ORIENTED_EDGE('',*,*,#1851,.T.);
#2293=ORIENTED_EDGE('',*,*,#1854,.F.);
#2294=ORIENTED_EDGE('',*,*,#1855,.F.);
#2295=ORIENTED_EDGE('',*,*,#1856,.T.);
#2296=ORIENTED_EDGE('',*,*,#1857,.F.);
#2297=ORIENTED_EDGE('',*,*,#1856,.F.);
#2298=ORIENTED_EDGE('',*,*,#1858,.F.);
#2299=ORIENTED_EDGE('',*,*,#1859,.F.);
#2300=ORIENTED_EDGE('',*,*,#1860,.F.);
#2301=ORIENTED_EDGE('',*,*,#1861,.T.);
#2302=ORIENTED_EDGE('',*,*,#1862,.F.);
#2303=ORIENTED_EDGE('',*,*,#1861,.F.);
#2304=ORIENTED_EDGE('',*,*,#1863,.F.);
#2305=ORIENTED_EDGE('',*,*,#1864,.F.);
#2306=ORIENTED_EDGE('',*,*,#1865,.F.);
#2307=ORIENTED_EDGE('',*,*,#1866,.T.);
#2308=ORIENTED_EDGE('',*,*,#1867,.F.);
#2309=ORIENTED_EDGE('',*,*,#1866,.F.);
#2310=ORIENTED_EDGE('',*,*,#1868,.F.);
#2311=ORIENTED_EDGE('',*,*,#1869,.F.);
#2312=ORIENTED_EDGE('',*,*,#1870,.T.);
#2313=ORIENTED_EDGE('',*,*,#1871,.F.);
#2314=ORIENTED_EDGE('',*,*,#1870,.F.);
#2315=ORIENTED_EDGE('',*,*,#1872,.F.);
#2316=ORIENTED_EDGE('',*,*,#1873,.T.);
#2317=ORIENTED_EDGE('',*,*,#1874,.F.);
#2318=ORIENTED_EDGE('',*,*,#1873,.F.);
#2319=ORIENTED_EDGE('',*,*,#1875,.F.);
#2320=ORIENTED_EDGE('',*,*,#1876,.T.);
#2321=ORIENTED_EDGE('',*,*,#1877,.F.);
#2322=ORIENTED_EDGE('',*,*,#1876,.F.);
#2323=ORIENTED_EDGE('',*,*,#1878,.F.);
#2324=ORIENTED_EDGE('',*,*,#1879,.T.);
#2325=ORIENTED_EDGE('',*,*,#1880,.F.);
#2326=ORIENTED_EDGE('',*,*,#1879,.F.);
#2327=ORIENTED_EDGE('',*,*,#1881,.F.);
#2328=ORIENTED_EDGE('',*,*,#1882,.T.);
#2329=ORIENTED_EDGE('',*,*,#1883,.F.);
#2330=ORIENTED_EDGE('',*,*,#1882,.F.);
#2331=ORIENTED_EDGE('',*,*,#1881,.T.);
#2332=ORIENTED_EDGE('',*,*,#1884,.F.);
#2333=ORIENTED_EDGE('',*,*,#1885,.F.);
#2334=ORIENTED_EDGE('',*,*,#1886,.T.);
#2335=ORIENTED_EDGE('',*,*,#1887,.F.);
#2336=ORIENTED_EDGE('',*,*,#1886,.F.);
#2337=ORIENTED_EDGE('',*,*,#1885,.T.);
#2338=ORIENTED_EDGE('',*,*,#1888,.F.);
#2339=ORIENTED_EDGE('',*,*,#1889,.F.);
#2340=ORIENTED_EDGE('',*,*,#1890,.T.);
#2341=ORIENTED_EDGE('',*,*,#1891,.F.);
#2342=ORIENTED_EDGE('',*,*,#1890,.F.);
#2343=ORIENTED_EDGE('',*,*,#1889,.T.);
#2344=ORIENTED_EDGE('',*,*,#1892,.F.);
#2345=ORIENTED_EDGE('',*,*,#1893,.F.);
#2346=ORIENTED_EDGE('',*,*,#1894,.T.);
#2347=ORIENTED_EDGE('',*,*,#1895,.T.);
#2348=ORIENTED_EDGE('',*,*,#1894,.F.);
#2349=ORIENTED_EDGE('',*,*,#1895,.F.);
#2350=ORIENTED_EDGE('',*,*,#1896,.F.);
#2351=ORIENTED_EDGE('',*,*,#1897,.F.);
#2352=ORIENTED_EDGE('',*,*,#1898,.T.);
#2353=ORIENTED_EDGE('',*,*,#1899,.T.);
#2354=ORIENTED_EDGE('',*,*,#1898,.F.);
#2355=ORIENTED_EDGE('',*,*,#1899,.F.);
#2356=ORIENTED_EDGE('',*,*,#1900,.F.);
#2357=ORIENTED_EDGE('',*,*,#1901,.F.);
#2358=ORIENTED_EDGE('',*,*,#1902,.T.);
#2359=ORIENTED_EDGE('',*,*,#1903,.T.);
#2360=ORIENTED_EDGE('',*,*,#1902,.F.);
#2361=ORIENTED_EDGE('',*,*,#1903,.F.);
#2362=ORIENTED_EDGE('',*,*,#1904,.F.);
#2363=ORIENTED_EDGE('',*,*,#1896,.T.);
#2364=ORIENTED_EDGE('',*,*,#1905,.T.);
#2365=ORIENTED_EDGE('',*,*,#1855,.T.);
#2366=ORIENTED_EDGE('',*,*,#1854,.T.);
#2367=ORIENTED_EDGE('',*,*,#1906,.T.);
#2368=ORIENTED_EDGE('',*,*,#1828,.T.);
#2369=ORIENTED_EDGE('',*,*,#1827,.T.);
#2370=ORIENTED_EDGE('',*,*,#1907,.T.);
#2371=ORIENTED_EDGE('',*,*,#1884,.T.);
#2372=ORIENTED_EDGE('',*,*,#1907,.F.);
#2373=ORIENTED_EDGE('',*,*,#1831,.T.);
#2374=ORIENTED_EDGE('',*,*,#1906,.F.);
#2375=ORIENTED_EDGE('',*,*,#1858,.T.);
#2376=ORIENTED_EDGE('',*,*,#1905,.F.);
#2377=ORIENTED_EDGE('',*,*,#1900,.T.);
#2378=ORIENTED_EDGE('',*,*,#1908,.T.);
#2379=ORIENTED_EDGE('',*,*,#1860,.T.);
#2380=ORIENTED_EDGE('',*,*,#1859,.T.);
#2381=ORIENTED_EDGE('',*,*,#1909,.T.);
#2382=ORIENTED_EDGE('',*,*,#1833,.T.);
#2383=ORIENTED_EDGE('',*,*,#1832,.T.);
#2384=ORIENTED_EDGE('',*,*,#1910,.T.);
#2385=ORIENTED_EDGE('',*,*,#1888,.T.);
#2386=ORIENTED_EDGE('',*,*,#1910,.F.);
#2387=ORIENTED_EDGE('',*,*,#1836,.T.);
#2388=ORIENTED_EDGE('',*,*,#1909,.F.);
#2389=ORIENTED_EDGE('',*,*,#1863,.T.);
#2390=ORIENTED_EDGE('',*,*,#1908,.F.);
#2391=ORIENTED_EDGE('',*,*,#1904,.T.);
#2392=ORIENTED_EDGE('',*,*,#1911,.T.);
#2393=ORIENTED_EDGE('',*,*,#1865,.T.);
#2394=ORIENTED_EDGE('',*,*,#1864,.T.);
#2395=ORIENTED_EDGE('',*,*,#1912,.T.);
#2396=ORIENTED_EDGE('',*,*,#1838,.T.);
#2397=ORIENTED_EDGE('',*,*,#1837,.T.);
#2398=ORIENTED_EDGE('',*,*,#1913,.T.);
#2399=ORIENTED_EDGE('',*,*,#1892,.T.);
#2400=ORIENTED_EDGE('',*,*,#1913,.F.);
#2401=ORIENTED_EDGE('',*,*,#1841,.T.);
#2402=ORIENTED_EDGE('',*,*,#1912,.F.);
#2403=ORIENTED_EDGE('',*,*,#1868,.T.);
#2404=ORIENTED_EDGE('',*,*,#1911,.F.);
#2405=ORIENTED_EDGE('',*,*,#1914,.T.);
#2406=ORIENTED_EDGE('',*,*,#1915,.T.);
#2407=ORIENTED_EDGE('',*,*,#1916,.F.);
#2408=ORIENTED_EDGE('',*,*,#1917,.F.);
#2409=ORIENTED_EDGE('',*,*,#1918,.T.);
#2410=ORIENTED_EDGE('',*,*,#1917,.T.);
#2411=ORIENTED_EDGE('',*,*,#1919,.F.);
#2412=ORIENTED_EDGE('',*,*,#1920,.F.);
#2413=ORIENTED_EDGE('',*,*,#1891,.T.);
#2414=ORIENTED_EDGE('',*,*,#1887,.T.);
#2415=ORIENTED_EDGE('',*,*,#1883,.T.);
#2416=ORIENTED_EDGE('',*,*,#1921,.T.);
#2417=ORIENTED_EDGE('',*,*,#1920,.T.);
#2418=ORIENTED_EDGE('',*,*,#1922,.F.);
#2419=ORIENTED_EDGE('',*,*,#1923,.F.);
#2420=ORIENTED_EDGE('',*,*,#1924,.T.);
#2421=ORIENTED_EDGE('',*,*,#1923,.T.);
#2422=ORIENTED_EDGE('',*,*,#1925,.F.);
#2423=ORIENTED_EDGE('',*,*,#1915,.F.);
#2424=ORIENTED_EDGE('',*,*,#1901,.T.);
#2425=ORIENTED_EDGE('',*,*,#1897,.T.);
#2426=ORIENTED_EDGE('',*,*,#1893,.T.);
#2427=ORIENTED_EDGE('',*,*,#1925,.T.);
#2428=ORIENTED_EDGE('',*,*,#1922,.T.);
#2429=ORIENTED_EDGE('',*,*,#1919,.T.);
#2430=ORIENTED_EDGE('',*,*,#1916,.T.);
#2431=ORIENTED_EDGE('',*,*,#1830,.T.);
#2432=ORIENTED_EDGE('',*,*,#1835,.T.);
#2433=ORIENTED_EDGE('',*,*,#1840,.T.);
#2434=ORIENTED_EDGE('',*,*,#1857,.T.);
#2435=ORIENTED_EDGE('',*,*,#1862,.T.);
#2436=ORIENTED_EDGE('',*,*,#1867,.T.);
#2437=ORIENTED_EDGE('',*,*,#1871,.T.);
#2438=ORIENTED_EDGE('',*,*,#1874,.T.);
#2439=ORIENTED_EDGE('',*,*,#1877,.T.);
#2440=ORIENTED_EDGE('',*,*,#1880,.T.);
#2441=ORIENTED_EDGE('',*,*,#1853,.T.);
#2442=ORIENTED_EDGE('',*,*,#1850,.T.);
#2443=ORIENTED_EDGE('',*,*,#1847,.T.);
#2444=ORIENTED_EDGE('',*,*,#1844,.T.);
#2445=ORIENTED_EDGE('',*,*,#1826,.T.);
#2446=ORIENTED_EDGE('',*,*,#1823,.T.);
#2447=ORIENTED_EDGE('',*,*,#1820,.T.);
#2448=ORIENTED_EDGE('',*,*,#1817,.T.);
#2449=ORIENTED_EDGE('',*,*,#1924,.F.);
#2450=ORIENTED_EDGE('',*,*,#1914,.F.);
#2451=ORIENTED_EDGE('',*,*,#1918,.F.);
#2452=ORIENTED_EDGE('',*,*,#1921,.F.);
#2453=ORIENTED_EDGE('',*,*,#1869,.T.);
#2454=ORIENTED_EDGE('',*,*,#1872,.T.);
#2455=ORIENTED_EDGE('',*,*,#1875,.T.);
#2456=ORIENTED_EDGE('',*,*,#1878,.T.);
#3075=CYLINDRICAL_SURFACE('',#3506,0.165);
#3076=CYLINDRICAL_SURFACE('',#3510,0.165);
#3077=CYLINDRICAL_SURFACE('',#3514,0.165);
#3078=CYLINDRICAL_SURFACE('',#3518,0.165);
#3079=CYLINDRICAL_SURFACE('',#3522,0.2);
#3080=CYLINDRICAL_SURFACE('',#3524,0.2);
#3081=CYLINDRICAL_SURFACE('',#3526,0.2);
#3082=CYLINDRICAL_SURFACE('',#3528,0.165);
#3083=CYLINDRICAL_SURFACE('',#3532,0.165);
#3084=CYLINDRICAL_SURFACE('',#3536,0.165);
#3085=CYLINDRICAL_SURFACE('',#3540,0.165);
#3086=CYLINDRICAL_SURFACE('',#3544,0.2);
#3087=CYLINDRICAL_SURFACE('',#3546,0.2);
#3088=CYLINDRICAL_SURFACE('',#3548,0.2);
#3089=CYLINDRICAL_SURFACE('',#3550,0.33);
#3090=CYLINDRICAL_SURFACE('',#3553,0.33);
#3091=CYLINDRICAL_SURFACE('',#3556,0.33);
#3092=CYLINDRICAL_SURFACE('',#3559,0.33);
#3093=CYLINDRICAL_SURFACE('',#3562,0.685);
#3094=CYLINDRICAL_SURFACE('',#3567,0.685);
#3095=CYLINDRICAL_SURFACE('',#3572,0.685);
#3096=CYLINDRICAL_SURFACE('',#3577,0.685);
#3097=CYLINDRICAL_SURFACE('',#3582,0.685);
#3098=CYLINDRICAL_SURFACE('',#3587,0.685);
#3099=CYLINDRICAL_SURFACE('',#3592,0.3);
#3100=CYLINDRICAL_SURFACE('',#3593,0.3);
#3101=CYLINDRICAL_SURFACE('',#3594,0.3);
#3159=ADVANCED_FACE('',(#386),#3075,.F.);
#3160=ADVANCED_FACE('',(#387),#277,.T.);
#3161=ADVANCED_FACE('',(#388),#3076,.F.);
#3162=ADVANCED_FACE('',(#389),#278,.T.);
#3163=ADVANCED_FACE('',(#390),#3077,.F.);
#3164=ADVANCED_FACE('',(#391),#279,.T.);
#3165=ADVANCED_FACE('',(#392),#3078,.F.);
#3166=ADVANCED_FACE('',(#393),#280,.T.);
#3167=ADVANCED_FACE('',(#394),#3079,.F.);
#3168=ADVANCED_FACE('',(#395),#3080,.F.);
#3169=ADVANCED_FACE('',(#396),#3081,.F.);
#3170=ADVANCED_FACE('',(#397),#3082,.F.);
#3171=ADVANCED_FACE('',(#398),#281,.T.);
#3172=ADVANCED_FACE('',(#399),#3083,.F.);
#3173=ADVANCED_FACE('',(#400),#282,.T.);
#3174=ADVANCED_FACE('',(#401),#3084,.F.);
#3175=ADVANCED_FACE('',(#402),#283,.T.);
#3176=ADVANCED_FACE('',(#403),#3085,.F.);
#3177=ADVANCED_FACE('',(#404),#284,.T.);
#3178=ADVANCED_FACE('',(#405),#3086,.F.);
#3179=ADVANCED_FACE('',(#406),#3087,.F.);
#3180=ADVANCED_FACE('',(#407),#3088,.F.);
#3181=ADVANCED_FACE('',(#408),#3089,.F.);
#3182=ADVANCED_FACE('',(#409),#3090,.F.);
#3183=ADVANCED_FACE('',(#410),#3091,.F.);
#3184=ADVANCED_FACE('',(#411),#3092,.F.);
#3185=ADVANCED_FACE('',(#412),#3093,.F.);
#3186=ADVANCED_FACE('',(#413,#142),#285,.T.);
#3187=ADVANCED_FACE('',(#414),#3094,.F.);
#3188=ADVANCED_FACE('',(#415,#143),#286,.T.);
#3189=ADVANCED_FACE('',(#416),#3095,.F.);
#3190=ADVANCED_FACE('',(#417,#144),#287,.T.);
#3191=ADVANCED_FACE('',(#418),#3096,.F.);
#3192=ADVANCED_FACE('',(#419,#145),#288,.F.);
#3193=ADVANCED_FACE('',(#420),#3097,.F.);
#3194=ADVANCED_FACE('',(#421,#146),#289,.F.);
#3195=ADVANCED_FACE('',(#422),#3098,.F.);
#3196=ADVANCED_FACE('',(#423,#147),#290,.F.);
#3197=ADVANCED_FACE('',(#424),#3099,.F.);
#3198=ADVANCED_FACE('',(#425),#3100,.F.);
#3199=ADVANCED_FACE('',(#426),#3101,.F.);
#3200=ADVANCED_FACE('',(#427),#291,.T.);
#3201=ADVANCED_FACE('',(#428,#148,#149,#150),#292,.T.);
#3202=ADVANCED_FACE('',(#429),#293,.T.);
#3203=ADVANCED_FACE('',(#430,#151,#152,#153),#294,.T.);
#3204=ADVANCED_FACE('',(#431,#154,#155,#156,#157,#158,#159,#160,#161,#162,
#163,#164,#165,#166,#167,#168,#169,#170,#171),#295,.T.);
#3205=ADVANCED_FACE('',(#432,#172,#173,#174,#175),#296,.F.);
#3358=CLOSED_SHELL('',(#3159,#3160,#3161,#3162,#3163,#3164,#3165,#3166,
#3167,#3168,#3169,#3170,#3171,#3172,#3173,#3174,#3175,#3176,#3177,#3178,
#3179,#3180,#3181,#3182,#3183,#3184,#3185,#3186,#3187,#3188,#3189,#3190,
#3191,#3192,#3193,#3194,#3195,#3196,#3197,#3198,#3199,#3200,#3201,#3202,
#3203,#3204,#3205));
#3505=AXIS2_PLACEMENT_3D('',#4942,#3907,#3908);
#3506=AXIS2_PLACEMENT_3D('',#4943,#3909,#3910);
#3507=AXIS2_PLACEMENT_3D('',#4945,#3911,#3912);
#3508=AXIS2_PLACEMENT_3D('',#4948,#3914,#3915);
#3509=AXIS2_PLACEMENT_3D('',#4949,#3916,#3917);
#3510=AXIS2_PLACEMENT_3D('',#4950,#3918,#3919);
#3511=AXIS2_PLACEMENT_3D('',#4952,#3920,#3921);
#3512=AXIS2_PLACEMENT_3D('',#4955,#3923,#3924);
#3513=AXIS2_PLACEMENT_3D('',#4956,#3925,#3926);
#3514=AXIS2_PLACEMENT_3D('',#4957,#3927,#3928);
#3515=AXIS2_PLACEMENT_3D('',#4959,#3929,#3930);
#3516=AXIS2_PLACEMENT_3D('',#4962,#3932,#3933);
#3517=AXIS2_PLACEMENT_3D('',#4963,#3934,#3935);
#3518=AXIS2_PLACEMENT_3D('',#4964,#3936,#3937);
#3519=AXIS2_PLACEMENT_3D('',#4966,#3938,#3939);
#3520=AXIS2_PLACEMENT_3D('',#4969,#3941,#3942);
#3521=AXIS2_PLACEMENT_3D('',#4970,#3943,#3944);
#3522=AXIS2_PLACEMENT_3D('',#4971,#3945,#3946);
#3523=AXIS2_PLACEMENT_3D('',#4997,#3948,#3949);
#3524=AXIS2_PLACEMENT_3D('',#5016,#3950,#3951);
#3525=AXIS2_PLACEMENT_3D('',#5042,#3953,#3954);
#3526=AXIS2_PLACEMENT_3D('',#5061,#3955,#3956);
#3527=AXIS2_PLACEMENT_3D('',#5087,#3958,#3959);
#3528=AXIS2_PLACEMENT_3D('',#5106,#3960,#3961);
#3529=AXIS2_PLACEMENT_3D('',#5108,#3962,#3963);
#3530=AXIS2_PLACEMENT_3D('',#5111,#3965,#3966);
#3531=AXIS2_PLACEMENT_3D('',#5112,#3967,#3968);
#3532=AXIS2_PLACEMENT_3D('',#5113,#3969,#3970);
#3533=AXIS2_PLACEMENT_3D('',#5115,#3971,#3972);
#3534=AXIS2_PLACEMENT_3D('',#5118,#3974,#3975);
#3535=AXIS2_PLACEMENT_3D('',#5119,#3976,#3977);
#3536=AXIS2_PLACEMENT_3D('',#5120,#3978,#3979);
#3537=AXIS2_PLACEMENT_3D('',#5122,#3980,#3981);
#3538=AXIS2_PLACEMENT_3D('',#5125,#3983,#3984);
#3539=AXIS2_PLACEMENT_3D('',#5126,#3985,#3986);
#3540=AXIS2_PLACEMENT_3D('',#5127,#3987,#3988);
#3541=AXIS2_PLACEMENT_3D('',#5129,#3989,#3990);
#3542=AXIS2_PLACEMENT_3D('',#5132,#3992,#3993);
#3543=AXIS2_PLACEMENT_3D('',#5133,#3994,#3995);
#3544=AXIS2_PLACEMENT_3D('',#5134,#3996,#3997);
#3545=AXIS2_PLACEMENT_3D('',#5160,#3999,#4000);
#3546=AXIS2_PLACEMENT_3D('',#5179,#4001,#4002);
#3547=AXIS2_PLACEMENT_3D('',#5205,#4004,#4005);
#3548=AXIS2_PLACEMENT_3D('',#5224,#4006,#4007);
#3549=AXIS2_PLACEMENT_3D('',#5250,#4009,#4010);
#3550=AXIS2_PLACEMENT_3D('',#5269,#4011,#4012);
#3551=AXIS2_PLACEMENT_3D('',#5271,#4013,#4014);
#3552=AXIS2_PLACEMENT_3D('',#5274,#4016,#4017);
#3553=AXIS2_PLACEMENT_3D('',#5275,#4018,#4019);
#3554=AXIS2_PLACEMENT_3D('',#5277,#4020,#4021);
#3555=AXIS2_PLACEMENT_3D('',#5280,#4023,#4024);
#3556=AXIS2_PLACEMENT_3D('',#5281,#4025,#4026);
#3557=AXIS2_PLACEMENT_3D('',#5283,#4027,#4028);
#3558=AXIS2_PLACEMENT_3D('',#5286,#4030,#4031);
#3559=AXIS2_PLACEMENT_3D('',#5287,#4032,#4033);
#3560=AXIS2_PLACEMENT_3D('',#5289,#4034,#4035);
#3561=AXIS2_PLACEMENT_3D('',#5292,#4037,#4038);
#3562=AXIS2_PLACEMENT_3D('',#5293,#4039,#4040);
#3563=AXIS2_PLACEMENT_3D('',#5295,#4041,#4042);
#3564=AXIS2_PLACEMENT_3D('',#5298,#4044,#4045);
#3565=AXIS2_PLACEMENT_3D('',#5299,#4046,#4047);
#3566=AXIS2_PLACEMENT_3D('',#5301,#4048,#4049);
#3567=AXIS2_PLACEMENT_3D('',#5302,#4050,#4051);
#3568=AXIS2_PLACEMENT_3D('',#5304,#4052,#4053);
#3569=AXIS2_PLACEMENT_3D('',#5307,#4055,#4056);
#3570=AXIS2_PLACEMENT_3D('',#5308,#4057,#4058);
#3571=AXIS2_PLACEMENT_3D('',#5310,#4059,#4060);
#3572=AXIS2_PLACEMENT_3D('',#5311,#4061,#4062);
#3573=AXIS2_PLACEMENT_3D('',#5313,#4063,#4064);
#3574=AXIS2_PLACEMENT_3D('',#5316,#4066,#4067);
#3575=AXIS2_PLACEMENT_3D('',#5317,#4068,#4069);
#3576=AXIS2_PLACEMENT_3D('',#5319,#4070,#4071);
#3577=AXIS2_PLACEMENT_3D('',#5320,#4072,#4073);
#3578=AXIS2_PLACEMENT_3D('',#5322,#4074,#4075);
#3579=AXIS2_PLACEMENT_3D('',#5325,#4077,#4078);
#3580=AXIS2_PLACEMENT_3D('',#5326,#4079,#4080);
#3581=AXIS2_PLACEMENT_3D('',#5328,#4081,#4082);
#3582=AXIS2_PLACEMENT_3D('',#5329,#4083,#4084);
#3583=AXIS2_PLACEMENT_3D('',#5331,#4085,#4086);
#3584=AXIS2_PLACEMENT_3D('',#5334,#4088,#4089);
#3585=AXIS2_PLACEMENT_3D('',#5335,#4090,#4091);
#3586=AXIS2_PLACEMENT_3D('',#5337,#4092,#4093);
#3587=AXIS2_PLACEMENT_3D('',#5338,#4094,#4095);
#3588=AXIS2_PLACEMENT_3D('',#5340,#4096,#4097);
#3589=AXIS2_PLACEMENT_3D('',#5343,#4099,#4100);
#3590=AXIS2_PLACEMENT_3D('',#5344,#4101,#4102);
#3591=AXIS2_PLACEMENT_3D('',#5346,#4103,#4104);
#3592=AXIS2_PLACEMENT_3D('',#5347,#4105,#4106);
#3593=AXIS2_PLACEMENT_3D('',#5351,#4110,#4111);
#3594=AXIS2_PLACEMENT_3D('',#5355,#4115,#4116);
#3595=AXIS2_PLACEMENT_3D('',#5359,#4120,#4121);
#3596=AXIS2_PLACEMENT_3D('',#5368,#4126,#4127);
#3597=AXIS2_PLACEMENT_3D('',#5374,#4131,#4132);
#3598=AXIS2_PLACEMENT_3D('',#5380,#4136,#4137);
#3599=AXIS2_PLACEMENT_3D('',#5383,#4140,#4141);
#3600=AXIS2_PLACEMENT_3D('',#5384,#4142,#4143);
#3907=DIRECTION('axis',(0.,0.,1.));
#3908=DIRECTION('refdir',(1.,0.,0.));
#3909=DIRECTION('center_axis',(0.,0.,1.));
#3910=DIRECTION('ref_axis',(1.,0.,0.));
#3911=DIRECTION('center_axis',(0.,0.,1.));
#3912=DIRECTION('ref_axis',(1.,0.,0.));
#3913=DIRECTION('',(0.,0.,1.));
#3914=DIRECTION('center_axis',(0.,0.,-1.));
#3915=DIRECTION('ref_axis',(1.,0.,0.));
#3916=DIRECTION('center_axis',(0.,0.,1.));
#3917=DIRECTION('ref_axis',(1.,0.,0.));
#3918=DIRECTION('center_axis',(0.,0.,1.));
#3919=DIRECTION('ref_axis',(1.,0.,0.));
#3920=DIRECTION('center_axis',(0.,0.,1.));
#3921=DIRECTION('ref_axis',(1.,0.,0.));
#3922=DIRECTION('',(0.,0.,1.));
#3923=DIRECTION('center_axis',(0.,0.,-1.));
#3924=DIRECTION('ref_axis',(1.,0.,0.));
#3925=DIRECTION('center_axis',(0.,0.,1.));
#3926=DIRECTION('ref_axis',(1.,0.,0.));
#3927=DIRECTION('center_axis',(0.,0.,1.));
#3928=DIRECTION('ref_axis',(1.,0.,0.));
#3929=DIRECTION('center_axis',(0.,0.,1.));
#3930=DIRECTION('ref_axis',(1.,0.,0.));
#3931=DIRECTION('',(0.,0.,1.));
#3932=DIRECTION('center_axis',(0.,0.,-1.));
#3933=DIRECTION('ref_axis',(1.,0.,0.));
#3934=DIRECTION('center_axis',(0.,0.,1.));
#3935=DIRECTION('ref_axis',(1.,0.,0.));
#3936=DIRECTION('center_axis',(0.,0.,1.));
#3937=DIRECTION('ref_axis',(1.,0.,0.));
#3938=DIRECTION('center_axis',(0.,0.,1.));
#3939=DIRECTION('ref_axis',(1.,0.,0.));
#3940=DIRECTION('',(0.,0.,1.));
#3941=DIRECTION('center_axis',(0.,0.,-1.));
#3942=DIRECTION('ref_axis',(1.,0.,0.));
#3943=DIRECTION('center_axis',(0.,0.,1.));
#3944=DIRECTION('ref_axis',(1.,0.,0.));
#3945=DIRECTION('center_axis',(0.,0.,1.));
#3946=DIRECTION('ref_axis',(1.,0.,0.));
#3947=DIRECTION('',(0.,0.,1.));
#3948=DIRECTION('center_axis',(0.,0.,-1.));
#3949=DIRECTION('ref_axis',(1.,0.,0.));
#3950=DIRECTION('center_axis',(0.,0.,1.));
#3951=DIRECTION('ref_axis',(1.,0.,0.));
#3952=DIRECTION('',(0.,0.,1.));
#3953=DIRECTION('center_axis',(0.,0.,-1.));
#3954=DIRECTION('ref_axis',(1.,0.,0.));
#3955=DIRECTION('center_axis',(0.,0.,1.));
#3956=DIRECTION('ref_axis',(1.,0.,0.));
#3957=DIRECTION('',(0.,0.,1.));
#3958=DIRECTION('center_axis',(0.,0.,-1.));
#3959=DIRECTION('ref_axis',(1.,0.,0.));
#3960=DIRECTION('center_axis',(0.,0.,1.));
#3961=DIRECTION('ref_axis',(1.,0.,0.));
#3962=DIRECTION('center_axis',(0.,0.,1.));
#3963=DIRECTION('ref_axis',(1.,0.,0.));
#3964=DIRECTION('',(0.,0.,1.));
#3965=DIRECTION('center_axis',(0.,0.,-1.));
#3966=DIRECTION('ref_axis',(1.,0.,0.));
#3967=DIRECTION('center_axis',(0.,0.,1.));
#3968=DIRECTION('ref_axis',(1.,0.,0.));
#3969=DIRECTION('center_axis',(0.,0.,1.));
#3970=DIRECTION('ref_axis',(1.,0.,0.));
#3971=DIRECTION('center_axis',(0.,0.,1.));
#3972=DIRECTION('ref_axis',(1.,0.,0.));
#3973=DIRECTION('',(0.,0.,1.));
#3974=DIRECTION('center_axis',(0.,0.,-1.));
#3975=DIRECTION('ref_axis',(1.,0.,0.));
#3976=DIRECTION('center_axis',(0.,0.,1.));
#3977=DIRECTION('ref_axis',(1.,0.,0.));
#3978=DIRECTION('center_axis',(0.,0.,1.));
#3979=DIRECTION('ref_axis',(1.,0.,0.));
#3980=DIRECTION('center_axis',(0.,0.,1.));
#3981=DIRECTION('ref_axis',(1.,0.,0.));
#3982=DIRECTION('',(0.,0.,1.));
#3983=DIRECTION('center_axis',(0.,0.,-1.));
#3984=DIRECTION('ref_axis',(1.,0.,0.));
#3985=DIRECTION('center_axis',(0.,0.,1.));
#3986=DIRECTION('ref_axis',(1.,0.,0.));
#3987=DIRECTION('center_axis',(0.,0.,1.));
#3988=DIRECTION('ref_axis',(1.,0.,0.));
#3989=DIRECTION('center_axis',(0.,0.,1.));
#3990=DIRECTION('ref_axis',(1.,0.,0.));
#3991=DIRECTION('',(0.,0.,1.));
#3992=DIRECTION('center_axis',(0.,0.,-1.));
#3993=DIRECTION('ref_axis',(1.,0.,0.));
#3994=DIRECTION('center_axis',(0.,0.,1.));
#3995=DIRECTION('ref_axis',(1.,0.,0.));
#3996=DIRECTION('center_axis',(0.,0.,1.));
#3997=DIRECTION('ref_axis',(1.,0.,0.));
#3998=DIRECTION('',(0.,0.,1.));
#3999=DIRECTION('center_axis',(0.,0.,-1.));
#4000=DIRECTION('ref_axis',(1.,0.,0.));
#4001=DIRECTION('center_axis',(0.,0.,1.));
#4002=DIRECTION('ref_axis',(1.,0.,0.));
#4003=DIRECTION('',(0.,0.,1.));
#4004=DIRECTION('center_axis',(0.,0.,-1.));
#4005=DIRECTION('ref_axis',(1.,0.,0.));
#4006=DIRECTION('center_axis',(0.,0.,1.));
#4007=DIRECTION('ref_axis',(1.,0.,0.));
#4008=DIRECTION('',(0.,0.,1.));
#4009=DIRECTION('center_axis',(0.,0.,-1.));
#4010=DIRECTION('ref_axis',(1.,0.,0.));
#4011=DIRECTION('center_axis',(0.,0.,1.));
#4012=DIRECTION('ref_axis',(1.,0.,0.));
#4013=DIRECTION('center_axis',(0.,0.,1.));
#4014=DIRECTION('ref_axis',(1.,0.,0.));
#4015=DIRECTION('',(0.,0.,1.));
#4016=DIRECTION('center_axis',(0.,0.,-1.));
#4017=DIRECTION('ref_axis',(1.,0.,0.));
#4018=DIRECTION('center_axis',(0.,0.,1.));
#4019=DIRECTION('ref_axis',(1.,0.,0.));
#4020=DIRECTION('center_axis',(0.,0.,1.));
#4021=DIRECTION('ref_axis',(1.,0.,0.));
#4022=DIRECTION('',(0.,0.,1.));
#4023=DIRECTION('center_axis',(0.,0.,-1.));
#4024=DIRECTION('ref_axis',(1.,0.,0.));
#4025=DIRECTION('center_axis',(0.,0.,1.));
#4026=DIRECTION('ref_axis',(1.,0.,0.));
#4027=DIRECTION('center_axis',(0.,0.,1.));
#4028=DIRECTION('ref_axis',(1.,0.,0.));
#4029=DIRECTION('',(0.,0.,1.));
#4030=DIRECTION('center_axis',(0.,0.,-1.));
#4031=DIRECTION('ref_axis',(1.,0.,0.));
#4032=DIRECTION('center_axis',(0.,0.,1.));
#4033=DIRECTION('ref_axis',(1.,0.,0.));
#4034=DIRECTION('center_axis',(0.,0.,1.));
#4035=DIRECTION('ref_axis',(1.,0.,0.));
#4036=DIRECTION('',(0.,0.,1.));
#4037=DIRECTION('center_axis',(0.,0.,-1.));
#4038=DIRECTION('ref_axis',(1.,0.,0.));
#4039=DIRECTION('center_axis',(1.,0.,0.));
#4040=DIRECTION('ref_axis',(0.,0.,-1.));
#4041=DIRECTION('center_axis',(1.,0.,0.));
#4042=DIRECTION('ref_axis',(0.,0.,-1.));
#4043=DIRECTION('',(1.,0.,0.));
#4044=DIRECTION('center_axis',(-1.,0.,0.));
#4045=DIRECTION('ref_axis',(0.,0.,-1.));
#4046=DIRECTION('center_axis',(1.,0.,0.));
#4047=DIRECTION('ref_axis',(0.,0.,-1.));
#4048=DIRECTION('center_axis',(1.,0.,0.));
#4049=DIRECTION('ref_axis',(0.,0.,-1.));
#4050=DIRECTION('center_axis',(1.,0.,0.));
#4051=DIRECTION('ref_axis',(0.,0.,-1.));
#4052=DIRECTION('center_axis',(1.,0.,0.));
#4053=DIRECTION('ref_axis',(0.,0.,-1.));
#4054=DIRECTION('',(1.,0.,0.));
#4055=DIRECTION('center_axis',(-1.,0.,0.));
#4056=DIRECTION('ref_axis',(0.,0.,-1.));
#4057=DIRECTION('center_axis',(1.,0.,0.));
#4058=DIRECTION('ref_axis',(0.,0.,-1.));
#4059=DIRECTION('center_axis',(1.,0.,0.));
#4060=DIRECTION('ref_axis',(0.,0.,-1.));
#4061=DIRECTION('center_axis',(1.,0.,0.));
#4062=DIRECTION('ref_axis',(0.,0.,-1.));
#4063=DIRECTION('center_axis',(1.,0.,0.));
#4064=DIRECTION('ref_axis',(0.,0.,-1.));
#4065=DIRECTION('',(1.,0.,0.));
#4066=DIRECTION('center_axis',(-1.,0.,0.));
#4067=DIRECTION('ref_axis',(0.,0.,-1.));
#4068=DIRECTION('center_axis',(1.,0.,0.));
#4069=DIRECTION('ref_axis',(0.,0.,-1.));
#4070=DIRECTION('center_axis',(1.,0.,0.));
#4071=DIRECTION('ref_axis',(0.,0.,-1.));
#4072=DIRECTION('center_axis',(1.,0.,0.));
#4073=DIRECTION('ref_axis',(0.,0.,-1.));
#4074=DIRECTION('center_axis',(1.,0.,0.));
#4075=DIRECTION('ref_axis',(0.,0.,-1.));
#4076=DIRECTION('',(1.,0.,0.));
#4077=DIRECTION('center_axis',(1.,0.,0.));
#4078=DIRECTION('ref_axis',(0.,0.,-1.));
#4079=DIRECTION('center_axis',(1.,0.,0.));
#4080=DIRECTION('ref_axis',(0.,0.,-1.));
#4081=DIRECTION('center_axis',(-1.,0.,0.));
#4082=DIRECTION('ref_axis',(0.,0.,-1.));
#4083=DIRECTION('center_axis',(1.,0.,0.));
#4084=DIRECTION('ref_axis',(0.,0.,-1.));
#4085=DIRECTION('center_axis',(1.,0.,0.));
#4086=DIRECTION('ref_axis',(0.,0.,-1.));
#4087=DIRECTION('',(1.,0.,0.));
#4088=DIRECTION('center_axis',(1.,0.,0.));
#4089=DIRECTION('ref_axis',(0.,0.,-1.));
#4090=DIRECTION('center_axis',(1.,0.,0.));
#4091=DIRECTION('ref_axis',(0.,0.,-1.));
#4092=DIRECTION('center_axis',(-1.,0.,0.));
#4093=DIRECTION('ref_axis',(0.,0.,-1.));
#4094=DIRECTION('center_axis',(1.,0.,0.));
#4095=DIRECTION('ref_axis',(0.,0.,-1.));
#4096=DIRECTION('center_axis',(1.,0.,0.));
#4097=DIRECTION('ref_axis',(0.,0.,-1.));
#4098=DIRECTION('',(1.,0.,0.));
#4099=DIRECTION('center_axis',(1.,0.,0.));
#4100=DIRECTION('ref_axis',(0.,0.,-1.));
#4101=DIRECTION('center_axis',(1.,0.,0.));
#4102=DIRECTION('ref_axis',(0.,0.,-1.));
#4103=DIRECTION('center_axis',(-1.,0.,0.));
#4104=DIRECTION('ref_axis',(0.,0.,-1.));
#4105=DIRECTION('center_axis',(1.,0.,0.));
#4106=DIRECTION('ref_axis',(0.,0.,-1.));
#4107=DIRECTION('',(1.,0.,0.));
#4108=DIRECTION('',(1.,0.,0.));
#4109=DIRECTION('',(1.,0.,0.));
#4110=DIRECTION('center_axis',(1.,0.,0.));
#4111=DIRECTION('ref_axis',(0.,0.,-1.));
#4112=DIRECTION('',(1.,0.,0.));
#4113=DIRECTION('',(1.,0.,0.));
#4114=DIRECTION('',(1.,0.,0.));
#4115=DIRECTION('center_axis',(1.,0.,0.));
#4116=DIRECTION('ref_axis',(0.,0.,-1.));
#4117=DIRECTION('',(1.,0.,0.));
#4118=DIRECTION('',(1.,0.,0.));
#4119=DIRECTION('',(1.,0.,0.));
#4120=DIRECTION('center_axis',(0.,1.,0.));
#4121=DIRECTION('ref_axis',(-1.,0.,0.));
#4122=DIRECTION('',(-1.,0.,0.));
#4123=DIRECTION('',(0.,0.,1.));
#4124=DIRECTION('',(-1.,0.,0.));
#4125=DIRECTION('',(0.,0.,1.));
#4126=DIRECTION('center_axis',(1.,0.,0.));
#4127=DIRECTION('ref_axis',(0.,1.,0.));
#4128=DIRECTION('',(0.,1.,0.));
#4129=DIRECTION('',(0.,1.,0.));
#4130=DIRECTION('',(0.,0.,1.));
#4131=DIRECTION('center_axis',(0.,-1.,0.));
#4132=DIRECTION('ref_axis',(1.,0.,0.));
#4133=DIRECTION('',(1.,0.,0.));
#4134=DIRECTION('',(1.,0.,0.));
#4135=DIRECTION('',(0.,0.,1.));
#4136=DIRECTION('center_axis',(-1.,0.,0.));
#4137=DIRECTION('ref_axis',(0.,-1.,0.));
#4138=DIRECTION('',(0.,-1.,0.));
#4139=DIRECTION('',(0.,-1.,0.));
#4140=DIRECTION('center_axis',(0.,0.,1.));
#4141=DIRECTION('ref_axis',(1.,0.,0.));
#4142=DIRECTION('center_axis',(0.,0.,1.));
#4143=DIRECTION('ref_axis',(1.,0.,0.));
#4942=CARTESIAN_POINT('',(0.,0.,0.));
#4943=CARTESIAN_POINT('Origin',(5.7,-2.4,0.8));
#4944=CARTESIAN_POINT('',(5.535,-2.4,0.8));
#4945=CARTESIAN_POINT('Origin',(5.7,-2.4,0.8));
#4946=CARTESIAN_POINT('',(5.535,-2.4,2.));
#4947=CARTESIAN_POINT('',(5.535,-2.4,0.8));
#4948=CARTESIAN_POINT('Origin',(5.7,-2.4,2.));
#4949=CARTESIAN_POINT('Origin',(5.7,-2.4,0.8));
#4950=CARTESIAN_POINT('Origin',(2.3,2.4,0.8));
#4951=CARTESIAN_POINT('',(2.135,2.4,0.8));
#4952=CARTESIAN_POINT('Origin',(2.3,2.4,0.8));
#4953=CARTESIAN_POINT('',(2.135,2.4,2.));
#4954=CARTESIAN_POINT('',(2.135,2.4,0.8));
#4955=CARTESIAN_POINT('Origin',(2.3,2.4,2.));
#4956=CARTESIAN_POINT('Origin',(2.3,2.4,0.8));
#4957=CARTESIAN_POINT('Origin',(2.3,-2.4,0.8));
#4958=CARTESIAN_POINT('',(2.135,-2.4,0.8));
#4959=CARTESIAN_POINT('Origin',(2.3,-2.4,0.8));
#4960=CARTESIAN_POINT('',(2.135,-2.4,2.));
#4961=CARTESIAN_POINT('',(2.135,-2.4,0.8));
#4962=CARTESIAN_POINT('Origin',(2.3,-2.4,2.));
#4963=CARTESIAN_POINT('Origin',(2.3,-2.4,0.8));
#4964=CARTESIAN_POINT('Origin',(5.7,2.4,0.8));
#4965=CARTESIAN_POINT('',(5.535,2.4,0.8));
#4966=CARTESIAN_POINT('Origin',(5.7,2.4,0.8));
#4967=CARTESIAN_POINT('',(5.535,2.4,2.));
#4968=CARTESIAN_POINT('',(5.535,2.4,0.8));
#4969=CARTESIAN_POINT('Origin',(5.7,2.4,2.));
#4970=CARTESIAN_POINT('Origin',(5.7,2.4,0.8));
#4971=CARTESIAN_POINT('Origin',(4.,-1.5,0.9));
#4972=CARTESIAN_POINT('',(4.,-1.7,1.22360679774998));
#4973=CARTESIAN_POINT('',(4.2,-1.5,1.3));
#4974=CARTESIAN_POINT('Ctrl Pts',(4.,-1.7,1.22360679774998));
#4975=CARTESIAN_POINT('Ctrl Pts',(4.02630182346442,-1.7,1.22360679774998));
#4976=CARTESIAN_POINT('Ctrl Pts',(4.05333179602069,-1.69456887761607,1.22872056892082));
#4977=CARTESIAN_POINT('Ctrl Pts',(4.10213335089966,-1.67398313783528,1.24474475389314));
#4978=CARTESIAN_POINT('Ctrl Pts',(4.12402433525871,-1.6588183772159,1.25527603224183));
#4979=CARTESIAN_POINT('Ctrl Pts',(4.15862698590242,-1.62421572657219,1.27377192701083));
#4980=CARTESIAN_POINT('Ctrl Pts',(4.17391823287771,-1.6022830144367,1.28316729552365));
#4981=CARTESIAN_POINT('Ctrl Pts',(4.19462445314031,-1.55320424736513,1.29633569102376));
#4982=CARTESIAN_POINT('Ctrl Pts',(4.2,-1.52601246699667,1.3));
#4983=CARTESIAN_POINT('Ctrl Pts',(4.2,-1.5,1.3));
#4984=CARTESIAN_POINT('',(3.8,-1.5,1.3));
#4985=CARTESIAN_POINT('Ctrl Pts',(3.8,-1.5,1.3));
#4986=CARTESIAN_POINT('Ctrl Pts',(3.8,-1.52601246699667,1.3));
#4987=CARTESIAN_POINT('Ctrl Pts',(3.80537554685969,-1.55320424736513,1.29633569102376));
#4988=CARTESIAN_POINT('Ctrl Pts',(3.82608176712229,-1.6022830144367,1.28316729552365));
#4989=CARTESIAN_POINT('Ctrl Pts',(3.84137301409757,-1.62421572657219,1.27377192701083));
#4990=CARTESIAN_POINT('Ctrl Pts',(3.87597566474129,-1.6588183772159,1.25527603224183));
#4991=CARTESIAN_POINT('Ctrl Pts',(3.89786664910035,-1.67398313783528,1.24474475389314));
#4992=CARTESIAN_POINT('Ctrl Pts',(3.94666820397931,-1.69456887761607,1.22872056892082));
#4993=CARTESIAN_POINT('Ctrl Pts',(3.97369817653558,-1.7,1.22360679774998));
#4994=CARTESIAN_POINT('Ctrl Pts',(4.,-1.7,1.22360679774998));
#4995=CARTESIAN_POINT('',(3.8,-1.5,2.));
#4996=CARTESIAN_POINT('',(3.8,-1.5,0.9));
#4997=CARTESIAN_POINT('Origin',(4.,-1.5,2.));
#4998=CARTESIAN_POINT('Ctrl Pts',(4.2,-1.5,1.3));
#4999=CARTESIAN_POINT('Ctrl Pts',(4.2,-1.47398753300333,1.3));
#5000=CARTESIAN_POINT('Ctrl Pts',(4.19462445314031,-1.44679575263487,1.29633569102376));
#5001=CARTESIAN_POINT('Ctrl Pts',(4.17391823287771,-1.3977169855633,1.28316729552365));
#5002=CARTESIAN_POINT('Ctrl Pts',(4.15862698590242,-1.37578427342781,1.27377192701083));
#5003=CARTESIAN_POINT('Ctrl Pts',(4.12402433525871,-1.3411816227841,1.25527603224183));
#5004=CARTESIAN_POINT('Ctrl Pts',(4.10213335089966,-1.32601686216472,1.24474475389314));
#5005=CARTESIAN_POINT('Ctrl Pts',(4.05333179602069,-1.30543112238393,1.22872056892082));
#5006=CARTESIAN_POINT('Ctrl Pts',(4.02630182346442,-1.3,1.22360679774998));
#5007=CARTESIAN_POINT('Ctrl Pts',(3.97369817653558,-1.3,1.22360679774998));
#5008=CARTESIAN_POINT('Ctrl Pts',(3.94666820397931,-1.30543112238393,1.22872056892082));
#5009=CARTESIAN_POINT('Ctrl Pts',(3.89786664910035,-1.32601686216472,1.24474475389314));
#5010=CARTESIAN_POINT('Ctrl Pts',(3.87597566474129,-1.3411816227841,1.25527603224183));
#5011=CARTESIAN_POINT('Ctrl Pts',(3.84137301409758,-1.37578427342781,1.27377192701083));
#5012=CARTESIAN_POINT('Ctrl Pts',(3.82608176712229,-1.3977169855633,1.28316729552365));
#5013=CARTESIAN_POINT('Ctrl Pts',(3.80537554685969,-1.44679575263487,1.29633569102376));
#5014=CARTESIAN_POINT('Ctrl Pts',(3.8,-1.47398753300333,1.3));
#5015=CARTESIAN_POINT('Ctrl Pts',(3.8,-1.5,1.3));
#5016=CARTESIAN_POINT('Origin',(4.,0.,0.9));
#5017=CARTESIAN_POINT('',(4.,-0.2,1.22360679774998));
#5018=CARTESIAN_POINT('',(4.2,-4.49191417939584E-18,1.3));
#5019=CARTESIAN_POINT('Ctrl Pts',(4.,-0.2,1.22360679774998));
#5020=CARTESIAN_POINT('Ctrl Pts',(4.02630182346442,-0.2,1.22360679774998));
#5021=CARTESIAN_POINT('Ctrl Pts',(4.05333179602069,-0.194568877616075,1.22872056892082));
#5022=CARTESIAN_POINT('Ctrl Pts',(4.10213335089966,-0.173983137835284,1.24474475389314));
#5023=CARTESIAN_POINT('Ctrl Pts',(4.12402433525871,-0.158818377215904,1.25527603224183));
#5024=CARTESIAN_POINT('Ctrl Pts',(4.15862698590242,-0.124215726572194,1.27377192701083));
#5025=CARTESIAN_POINT('Ctrl Pts',(4.17391823287771,-0.102283014436698,1.28316729552365));
#5026=CARTESIAN_POINT('Ctrl Pts',(4.19462445314031,-0.0532042473651346,
1.29633569102376));
#5027=CARTESIAN_POINT('Ctrl Pts',(4.2,-0.0260124669966693,1.3));
#5028=CARTESIAN_POINT('Ctrl Pts',(4.2,4.5102810375397E-17,1.3));
#5029=CARTESIAN_POINT('',(3.8,-6.08187253188241E-17,1.3));
#5030=CARTESIAN_POINT('Ctrl Pts',(3.8,-8.32667268468867E-17,1.3));
#5031=CARTESIAN_POINT('Ctrl Pts',(3.8,-0.0260124669966695,1.3));
#5032=CARTESIAN_POINT('Ctrl Pts',(3.80537554685969,-0.0532042473651335,
1.29633569102376));
#5033=CARTESIAN_POINT('Ctrl Pts',(3.82608176712229,-0.102283014436697,1.28316729552365));
#5034=CARTESIAN_POINT('Ctrl Pts',(3.84137301409758,-0.124215726572194,1.27377192701083));
#5035=CARTESIAN_POINT('Ctrl Pts',(3.87597566474129,-0.158818377215904,1.25527603224183));
#5036=CARTESIAN_POINT('Ctrl Pts',(3.89786664910035,-0.173983137835284,1.24474475389314));
#5037=CARTESIAN_POINT('Ctrl Pts',(3.94666820397931,-0.194568877616075,1.22872056892082));
#5038=CARTESIAN_POINT('Ctrl Pts',(3.97369817653558,-0.2,1.22360679774998));
#5039=CARTESIAN_POINT('Ctrl Pts',(4.,-0.2,1.22360679774998));
#5040=CARTESIAN_POINT('',(3.8,2.44929359829471E-17,2.));
#5041=CARTESIAN_POINT('',(3.8,-2.44929359829471E-17,0.9));
#5042=CARTESIAN_POINT('Origin',(4.,0.,2.));
#5043=CARTESIAN_POINT('Ctrl Pts',(4.2,2.77555756156289E-17,1.3));
#5044=CARTESIAN_POINT('Ctrl Pts',(4.2,0.0260124669966694,1.3));
#5045=CARTESIAN_POINT('Ctrl Pts',(4.19462445314031,0.0532042473651346,1.29633569102376));
#5046=CARTESIAN_POINT('Ctrl Pts',(4.17391823287771,0.102283014436698,1.28316729552365));
#5047=CARTESIAN_POINT('Ctrl Pts',(4.15862698590242,0.124215726572194,1.27377192701083));
#5048=CARTESIAN_POINT('Ctrl Pts',(4.12402433525871,0.158818377215904,1.25527603224183));
#5049=CARTESIAN_POINT('Ctrl Pts',(4.10213335089966,0.173983137835284,1.24474475389314));
#5050=CARTESIAN_POINT('Ctrl Pts',(4.05333179602069,0.194568877616075,1.22872056892082));
#5051=CARTESIAN_POINT('Ctrl Pts',(4.02630182346442,0.2,1.22360679774998));
#5052=CARTESIAN_POINT('Ctrl Pts',(3.97369817653558,0.2,1.22360679774998));
#5053=CARTESIAN_POINT('Ctrl Pts',(3.94666820397931,0.194568877616075,1.22872056892082));
#5054=CARTESIAN_POINT('Ctrl Pts',(3.89786664910035,0.173983137835284,1.24474475389314));
#5055=CARTESIAN_POINT('Ctrl Pts',(3.87597566474129,0.158818377215904,1.25527603224183));
#5056=CARTESIAN_POINT('Ctrl Pts',(3.84137301409758,0.124215726572194,1.27377192701083));
#5057=CARTESIAN_POINT('Ctrl Pts',(3.82608176712229,0.102283014436697,1.28316729552365));
#5058=CARTESIAN_POINT('Ctrl Pts',(3.80537554685969,0.0532042473651339,1.29633569102376));
#5059=CARTESIAN_POINT('Ctrl Pts',(3.8,0.0260124669966693,1.3));
#5060=CARTESIAN_POINT('Ctrl Pts',(3.8,-4.16333634234434E-17,1.3));
#5061=CARTESIAN_POINT('Origin',(4.,1.5,0.9));
#5062=CARTESIAN_POINT('',(4.,1.3,1.22360679774998));
#5063=CARTESIAN_POINT('',(4.2,1.5,1.3));
#5064=CARTESIAN_POINT('Ctrl Pts',(4.,1.3,1.22360679774998));
#5065=CARTESIAN_POINT('Ctrl Pts',(4.02630182346442,1.3,1.22360679774998));
#5066=CARTESIAN_POINT('Ctrl Pts',(4.05333179602069,1.30543112238393,1.22872056892082));
#5067=CARTESIAN_POINT('Ctrl Pts',(4.10213335089966,1.32601686216472,1.24474475389314));
#5068=CARTESIAN_POINT('Ctrl Pts',(4.12402433525871,1.3411816227841,1.25527603224183));
#5069=CARTESIAN_POINT('Ctrl Pts',(4.15862698590242,1.37578427342781,1.27377192701083));
#5070=CARTESIAN_POINT('Ctrl Pts',(4.17391823287771,1.3977169855633,1.28316729552365));
#5071=CARTESIAN_POINT('Ctrl Pts',(4.19462445314031,1.44679575263487,1.29633569102376));
#5072=CARTESIAN_POINT('Ctrl Pts',(4.2,1.47398753300333,1.3));
#5073=CARTESIAN_POINT('Ctrl Pts',(4.2,1.5,1.3));
#5074=CARTESIAN_POINT('',(3.8,1.5,1.3));
#5075=CARTESIAN_POINT('Ctrl Pts',(3.8,1.5,1.3));
#5076=CARTESIAN_POINT('Ctrl Pts',(3.8,1.47398753300333,1.3));
#5077=CARTESIAN_POINT('Ctrl Pts',(3.80537554685969,1.44679575263487,1.29633569102376));
#5078=CARTESIAN_POINT('Ctrl Pts',(3.82608176712229,1.3977169855633,1.28316729552365));
#5079=CARTESIAN_POINT('Ctrl Pts',(3.84137301409757,1.37578427342781,1.27377192701083));
#5080=CARTESIAN_POINT('Ctrl Pts',(3.87597566474129,1.3411816227841,1.25527603224183));
#5081=CARTESIAN_POINT('Ctrl Pts',(3.89786664910035,1.32601686216472,1.24474475389314));
#5082=CARTESIAN_POINT('Ctrl Pts',(3.94666820397931,1.30543112238393,1.22872056892082));
#5083=CARTESIAN_POINT('Ctrl Pts',(3.97369817653558,1.3,1.22360679774998));
#5084=CARTESIAN_POINT('Ctrl Pts',(4.,1.3,1.22360679774998));
#5085=CARTESIAN_POINT('',(3.8,1.5,2.));
#5086=CARTESIAN_POINT('',(3.8,1.5,0.9));
#5087=CARTESIAN_POINT('Origin',(4.,1.5,2.));
#5088=CARTESIAN_POINT('Ctrl Pts',(4.2,1.5,1.3));
#5089=CARTESIAN_POINT('Ctrl Pts',(4.2,1.52601246699667,1.3));
#5090=CARTESIAN_POINT('Ctrl Pts',(4.19462445314031,1.55320424736513,1.29633569102376));
#5091=CARTESIAN_POINT('Ctrl Pts',(4.17391823287771,1.6022830144367,1.28316729552365));
#5092=CARTESIAN_POINT('Ctrl Pts',(4.15862698590242,1.62421572657219,1.27377192701083));
#5093=CARTESIAN_POINT('Ctrl Pts',(4.12402433525871,1.6588183772159,1.25527603224183));
#5094=CARTESIAN_POINT('Ctrl Pts',(4.10213335089966,1.67398313783528,1.24474475389314));
#5095=CARTESIAN_POINT('Ctrl Pts',(4.05333179602069,1.69456887761607,1.22872056892082));
#5096=CARTESIAN_POINT('Ctrl Pts',(4.02630182346442,1.7,1.22360679774998));
#5097=CARTESIAN_POINT('Ctrl Pts',(3.97369817653558,1.7,1.22360679774998));
#5098=CARTESIAN_POINT('Ctrl Pts',(3.94666820397931,1.69456887761607,1.22872056892082));
#5099=CARTESIAN_POINT('Ctrl Pts',(3.89786664910035,1.67398313783528,1.24474475389314));
#5100=CARTESIAN_POINT('Ctrl Pts',(3.87597566474129,1.6588183772159,1.25527603224183));
#5101=CARTESIAN_POINT('Ctrl Pts',(3.84137301409758,1.62421572657219,1.27377192701083));
#5102=CARTESIAN_POINT('Ctrl Pts',(3.82608176712229,1.6022830144367,1.28316729552365));
#5103=CARTESIAN_POINT('Ctrl Pts',(3.80537554685969,1.55320424736513,1.29633569102376));
#5104=CARTESIAN_POINT('Ctrl Pts',(3.8,1.52601246699667,1.3));
#5105=CARTESIAN_POINT('Ctrl Pts',(3.8,1.5,1.3));
#5106=CARTESIAN_POINT('Origin',(-2.3,-2.4,0.8));
#5107=CARTESIAN_POINT('',(-2.465,-2.4,0.8));
#5108=CARTESIAN_POINT('Origin',(-2.3,-2.4,0.8));
#5109=CARTESIAN_POINT('',(-2.465,-2.4,2.));
#5110=CARTESIAN_POINT('',(-2.465,-2.4,0.8));
#5111=CARTESIAN_POINT('Origin',(-2.3,-2.4,2.));
#5112=CARTESIAN_POINT('Origin',(-2.3,-2.4,0.8));
#5113=CARTESIAN_POINT('Origin',(-5.7,2.4,0.8));
#5114=CARTESIAN_POINT('',(-5.865,2.4,0.8));
#5115=CARTESIAN_POINT('Origin',(-5.7,2.4,0.8));
#5116=CARTESIAN_POINT('',(-5.865,2.4,2.));
#5117=CARTESIAN_POINT('',(-5.865,2.4,0.8));
#5118=CARTESIAN_POINT('Origin',(-5.7,2.4,2.));
#5119=CARTESIAN_POINT('Origin',(-5.7,2.4,0.8));
#5120=CARTESIAN_POINT('Origin',(-5.7,-2.4,0.8));
#5121=CARTESIAN_POINT('',(-5.865,-2.4,0.8));
#5122=CARTESIAN_POINT('Origin',(-5.7,-2.4,0.8));
#5123=CARTESIAN_POINT('',(-5.865,-2.4,2.));
#5124=CARTESIAN_POINT('',(-5.865,-2.4,0.8));
#5125=CARTESIAN_POINT('Origin',(-5.7,-2.4,2.));
#5126=CARTESIAN_POINT('Origin',(-5.7,-2.4,0.8));
#5127=CARTESIAN_POINT('Origin',(-2.3,2.4,0.8));
#5128=CARTESIAN_POINT('',(-2.465,2.4,0.8));
#5129=CARTESIAN_POINT('Origin',(-2.3,2.4,0.8));
#5130=CARTESIAN_POINT('',(-2.465,2.4,2.));
#5131=CARTESIAN_POINT('',(-2.465,2.4,0.8));
#5132=CARTESIAN_POINT('Origin',(-2.3,2.4,2.));
#5133=CARTESIAN_POINT('Origin',(-2.3,2.4,0.8));
#5134=CARTESIAN_POINT('Origin',(-4.,-1.5,0.9));
#5135=CARTESIAN_POINT('',(-4.,-1.7,1.22360679774998));
#5136=CARTESIAN_POINT('',(-3.8,-1.5,1.3));
#5137=CARTESIAN_POINT('Ctrl Pts',(-4.,-1.7,1.22360679774998));
#5138=CARTESIAN_POINT('Ctrl Pts',(-3.97369817653558,-1.7,1.22360679774998));
#5139=CARTESIAN_POINT('Ctrl Pts',(-3.94666820397931,-1.69456887761608,1.22872056892082));
#5140=CARTESIAN_POINT('Ctrl Pts',(-3.89786664910035,-1.67398313783528,1.24474475389314));
#5141=CARTESIAN_POINT('Ctrl Pts',(-3.87597566474129,-1.6588183772159,1.25527603224183));
#5142=CARTESIAN_POINT('Ctrl Pts',(-3.84137301409758,-1.62421572657219,1.27377192701083));
#5143=CARTESIAN_POINT('Ctrl Pts',(-3.82608176712229,-1.6022830144367,1.28316729552365));
#5144=CARTESIAN_POINT('Ctrl Pts',(-3.80537554685969,-1.55320424736513,1.29633569102376));
#5145=CARTESIAN_POINT('Ctrl Pts',(-3.8,-1.52601246699667,1.3));
#5146=CARTESIAN_POINT('Ctrl Pts',(-3.8,-1.5,1.3));
#5147=CARTESIAN_POINT('',(-4.2,-1.5,1.3));
#5148=CARTESIAN_POINT('Ctrl Pts',(-4.2,-1.5,1.3));
#5149=CARTESIAN_POINT('Ctrl Pts',(-4.2,-1.52601246699667,1.3));
#5150=CARTESIAN_POINT('Ctrl Pts',(-4.19462445314031,-1.55320424736513,1.29633569102376));
#5151=CARTESIAN_POINT('Ctrl Pts',(-4.17391823287771,-1.6022830144367,1.28316729552365));
#5152=CARTESIAN_POINT('Ctrl Pts',(-4.15862698590242,-1.62421572657219,1.27377192701083));
#5153=CARTESIAN_POINT('Ctrl Pts',(-4.12402433525871,-1.6588183772159,1.25527603224183));
#5154=CARTESIAN_POINT('Ctrl Pts',(-4.10213335089965,-1.67398313783528,1.24474475389314));
#5155=CARTESIAN_POINT('Ctrl Pts',(-4.05333179602069,-1.69456887761608,1.22872056892082));
#5156=CARTESIAN_POINT('Ctrl Pts',(-4.02630182346442,-1.7,1.22360679774998));
#5157=CARTESIAN_POINT('Ctrl Pts',(-4.,-1.7,1.22360679774998));
#5158=CARTESIAN_POINT('',(-4.2,-1.5,2.));
#5159=CARTESIAN_POINT('',(-4.2,-1.5,0.9));
#5160=CARTESIAN_POINT('Origin',(-4.,-1.5,2.));
#5161=CARTESIAN_POINT('Ctrl Pts',(-3.8,-1.5,1.3));
#5162=CARTESIAN_POINT('Ctrl Pts',(-3.8,-1.47398753300333,1.3));
#5163=CARTESIAN_POINT('Ctrl Pts',(-3.80537554685969,-1.44679575263487,1.29633569102376));
#5164=CARTESIAN_POINT('Ctrl Pts',(-3.82608176712229,-1.3977169855633,1.28316729552365));
#5165=CARTESIAN_POINT('Ctrl Pts',(-3.84137301409758,-1.37578427342781,1.27377192701083));
#5166=CARTESIAN_POINT('Ctrl Pts',(-3.87597566474129,-1.3411816227841,1.25527603224183));
#5167=CARTESIAN_POINT('Ctrl Pts',(-3.89786664910035,-1.32601686216472,1.24474475389314));
#5168=CARTESIAN_POINT('Ctrl Pts',(-3.94666820397931,-1.30543112238392,1.22872056892082));
#5169=CARTESIAN_POINT('Ctrl Pts',(-3.97369817653558,-1.3,1.22360679774998));
#5170=CARTESIAN_POINT('Ctrl Pts',(-4.02630182346442,-1.3,1.22360679774998));
#5171=CARTESIAN_POINT('Ctrl Pts',(-4.05333179602069,-1.30543112238393,1.22872056892082));
#5172=CARTESIAN_POINT('Ctrl Pts',(-4.10213335089966,-1.32601686216472,1.24474475389314));
#5173=CARTESIAN_POINT('Ctrl Pts',(-4.12402433525871,-1.3411816227841,1.25527603224183));
#5174=CARTESIAN_POINT('Ctrl Pts',(-4.15862698590242,-1.37578427342781,1.27377192701083));
#5175=CARTESIAN_POINT('Ctrl Pts',(-4.17391823287771,-1.3977169855633,1.28316729552365));
#5176=CARTESIAN_POINT('Ctrl Pts',(-4.19462445314031,-1.44679575263487,1.29633569102376));
#5177=CARTESIAN_POINT('Ctrl Pts',(-4.2,-1.47398753300333,1.3));
#5178=CARTESIAN_POINT('Ctrl Pts',(-4.2,-1.5,1.3));
#5179=CARTESIAN_POINT('Origin',(-4.,0.,0.9));
#5180=CARTESIAN_POINT('',(-4.,-0.2,1.22360679774998));
#5181=CARTESIAN_POINT('',(-3.8,9.38587362841861E-18,1.3));
#5182=CARTESIAN_POINT('Ctrl Pts',(-4.,-0.2,1.22360679774998));
#5183=CARTESIAN_POINT('Ctrl Pts',(-3.97369817653558,-0.2,1.22360679774998));
#5184=CARTESIAN_POINT('Ctrl Pts',(-3.94666820397931,-0.194568877616075,
1.22872056892082));
#5185=CARTESIAN_POINT('Ctrl Pts',(-3.89786664910035,-0.173983137835284,
1.24474475389314));
#5186=CARTESIAN_POINT('Ctrl Pts',(-3.87597566474129,-0.158818377215904,
1.25527603224183));
#5187=CARTESIAN_POINT('Ctrl Pts',(-3.84137301409758,-0.124215726572194,
1.27377192701083));
#5188=CARTESIAN_POINT('Ctrl Pts',(-3.82608176712229,-0.102283014436697,
1.28316729552365));
#5189=CARTESIAN_POINT('Ctrl Pts',(-3.80537554685969,-0.053204247365134,
1.29633569102376));
#5190=CARTESIAN_POINT('Ctrl Pts',(-3.8,-0.0260124669966693,1.3));
#5191=CARTESIAN_POINT('Ctrl Pts',(-3.8,5.55111512312578E-17,1.3));
#5192=CARTESIAN_POINT('',(-4.2,-2.26548088473344E-17,1.3));
#5193=CARTESIAN_POINT('Ctrl Pts',(-4.2,-3.12250225675825E-17,1.3));
#5194=CARTESIAN_POINT('Ctrl Pts',(-4.2,-0.0260124669966694,1.3));
#5195=CARTESIAN_POINT('Ctrl Pts',(-4.19462445314031,-0.0532042473651348,
1.29633569102376));
#5196=CARTESIAN_POINT('Ctrl Pts',(-4.17391823287771,-0.102283014436698,
1.28316729552365));
#5197=CARTESIAN_POINT('Ctrl Pts',(-4.15862698590242,-0.124215726572194,
1.27377192701083));
#5198=CARTESIAN_POINT('Ctrl Pts',(-4.12402433525871,-0.158818377215904,
1.25527603224183));
#5199=CARTESIAN_POINT('Ctrl Pts',(-4.10213335089965,-0.173983137835285,
1.24474475389314));
#5200=CARTESIAN_POINT('Ctrl Pts',(-4.05333179602069,-0.194568877616075,
1.22872056892082));
#5201=CARTESIAN_POINT('Ctrl Pts',(-4.02630182346442,-0.2,1.22360679774998));
#5202=CARTESIAN_POINT('Ctrl Pts',(-4.,-0.2,1.22360679774998));
#5203=CARTESIAN_POINT('',(-4.2,2.44929359829471E-17,2.));
#5204=CARTESIAN_POINT('',(-4.2,-2.44929359829471E-17,0.9));
#5205=CARTESIAN_POINT('Origin',(-4.,0.,2.));
#5206=CARTESIAN_POINT('Ctrl Pts',(-3.8,5.55111512312578E-17,1.3));
#5207=CARTESIAN_POINT('Ctrl Pts',(-3.8,0.0260124669966694,1.3));
#5208=CARTESIAN_POINT('Ctrl Pts',(-3.80537554685969,0.053204247365134,1.29633569102376));
#5209=CARTESIAN_POINT('Ctrl Pts',(-3.82608176712229,0.102283014436697,1.28316729552365));
#5210=CARTESIAN_POINT('Ctrl Pts',(-3.84137301409758,0.124215726572194,1.27377192701083));
#5211=CARTESIAN_POINT('Ctrl Pts',(-3.87597566474129,0.158818377215904,1.25527603224183));
#5212=CARTESIAN_POINT('Ctrl Pts',(-3.89786664910035,0.173983137835284,1.24474475389314));
#5213=CARTESIAN_POINT('Ctrl Pts',(-3.94666820397931,0.194568877616075,1.22872056892082));
#5214=CARTESIAN_POINT('Ctrl Pts',(-3.97369817653558,0.2,1.22360679774998));
#5215=CARTESIAN_POINT('Ctrl Pts',(-4.02630182346442,0.2,1.22360679774998));
#5216=CARTESIAN_POINT('Ctrl Pts',(-4.05333179602069,0.194568877616075,1.22872056892082));
#5217=CARTESIAN_POINT('Ctrl Pts',(-4.10213335089966,0.173983137835284,1.24474475389314));
#5218=CARTESIAN_POINT('Ctrl Pts',(-4.12402433525871,0.158818377215904,1.25527603224183));
#5219=CARTESIAN_POINT('Ctrl Pts',(-4.15862698590242,0.124215726572194,1.27377192701083));
#5220=CARTESIAN_POINT('Ctrl Pts',(-4.17391823287771,0.102283014436697,1.28316729552365));
#5221=CARTESIAN_POINT('Ctrl Pts',(-4.19462445314031,0.0532042473651342,
1.29633569102376));
#5222=CARTESIAN_POINT('Ctrl Pts',(-4.2,0.0260124669966694,1.3));
#5223=CARTESIAN_POINT('Ctrl Pts',(-4.2,3.46944695195361E-18,1.3));
#5224=CARTESIAN_POINT('Origin',(-4.,1.5,0.9));
#5225=CARTESIAN_POINT('',(-4.,1.3,1.22360679774998));
#5226=CARTESIAN_POINT('',(-3.8,1.5,1.3));
#5227=CARTESIAN_POINT('Ctrl Pts',(-4.,1.3,1.22360679774998));
#5228=CARTESIAN_POINT('Ctrl Pts',(-3.97369817653558,1.3,1.22360679774998));
#5229=CARTESIAN_POINT('Ctrl Pts',(-3.94666820397931,1.30543112238392,1.22872056892082));
#5230=CARTESIAN_POINT('Ctrl Pts',(-3.89786664910035,1.32601686216472,1.24474475389314));
#5231=CARTESIAN_POINT('Ctrl Pts',(-3.87597566474129,1.3411816227841,1.25527603224183));
#5232=CARTESIAN_POINT('Ctrl Pts',(-3.84137301409758,1.37578427342781,1.27377192701083));
#5233=CARTESIAN_POINT('Ctrl Pts',(-3.82608176712229,1.3977169855633,1.28316729552365));
#5234=CARTESIAN_POINT('Ctrl Pts',(-3.80537554685969,1.44679575263487,1.29633569102376));
#5235=CARTESIAN_POINT('Ctrl Pts',(-3.8,1.47398753300333,1.3));
#5236=CARTESIAN_POINT('Ctrl Pts',(-3.8,1.5,1.3));
#5237=CARTESIAN_POINT('',(-4.2,1.5,1.3));
#5238=CARTESIAN_POINT('Ctrl Pts',(-4.2,1.5,1.3));
#5239=CARTESIAN_POINT('Ctrl Pts',(-4.2,1.47398753300333,1.3));
#5240=CARTESIAN_POINT('Ctrl Pts',(-4.19462445314031,1.44679575263487,1.29633569102376));
#5241=CARTESIAN_POINT('Ctrl Pts',(-4.17391823287771,1.3977169855633,1.28316729552365));
#5242=CARTESIAN_POINT('Ctrl Pts',(-4.15862698590242,1.37578427342781,1.27377192701083));
#5243=CARTESIAN_POINT('Ctrl Pts',(-4.12402433525871,1.3411816227841,1.25527603224183));
#5244=CARTESIAN_POINT('Ctrl Pts',(-4.10213335089965,1.32601686216472,1.24474475389314));
#5245=CARTESIAN_POINT('Ctrl Pts',(-4.05333179602069,1.30543112238392,1.22872056892082));
#5246=CARTESIAN_POINT('Ctrl Pts',(-4.02630182346442,1.3,1.22360679774998));
#5247=CARTESIAN_POINT('Ctrl Pts',(-4.,1.3,1.22360679774998));
#5248=CARTESIAN_POINT('',(-4.2,1.5,2.));
#5249=CARTESIAN_POINT('',(-4.2,1.5,0.9));
#5250=CARTESIAN_POINT('Origin',(-4.,1.5,2.));
#5251=CARTESIAN_POINT('Ctrl Pts',(-3.8,1.5,1.3));
#5252=CARTESIAN_POINT('Ctrl Pts',(-3.8,1.52601246699667,1.3));
#5253=CARTESIAN_POINT('Ctrl Pts',(-3.80537554685969,1.55320424736513,1.29633569102376));
#5254=CARTESIAN_POINT('Ctrl Pts',(-3.82608176712229,1.6022830144367,1.28316729552365));
#5255=CARTESIAN_POINT('Ctrl Pts',(-3.84137301409758,1.62421572657219,1.27377192701083));
#5256=CARTESIAN_POINT('Ctrl Pts',(-3.87597566474129,1.6588183772159,1.25527603224183));
#5257=CARTESIAN_POINT('Ctrl Pts',(-3.89786664910035,1.67398313783528,1.24474475389314));
#5258=CARTESIAN_POINT('Ctrl Pts',(-3.94666820397931,1.69456887761608,1.22872056892082));
#5259=CARTESIAN_POINT('Ctrl Pts',(-3.97369817653558,1.7,1.22360679774998));
#5260=CARTESIAN_POINT('Ctrl Pts',(-4.02630182346442,1.7,1.22360679774998));
#5261=CARTESIAN_POINT('Ctrl Pts',(-4.05333179602069,1.69456887761607,1.22872056892082));
#5262=CARTESIAN_POINT('Ctrl Pts',(-4.10213335089966,1.67398313783528,1.24474475389314));
#5263=CARTESIAN_POINT('Ctrl Pts',(-4.12402433525871,1.6588183772159,1.25527603224183));
#5264=CARTESIAN_POINT('Ctrl Pts',(-4.15862698590242,1.62421572657219,1.27377192701083));
#5265=CARTESIAN_POINT('Ctrl Pts',(-4.17391823287771,1.6022830144367,1.28316729552365));
#5266=CARTESIAN_POINT('Ctrl Pts',(-4.19462445314031,1.55320424736513,1.29633569102376));
#5267=CARTESIAN_POINT('Ctrl Pts',(-4.2,1.52601246699667,1.3));
#5268=CARTESIAN_POINT('Ctrl Pts',(-4.2,1.5,1.3));
#5269=CARTESIAN_POINT('Origin',(7.,-3.2,-0.1));
#5270=CARTESIAN_POINT('',(6.67,-3.2,0.));
#5271=CARTESIAN_POINT('Origin',(7.,-3.2,0.));
#5272=CARTESIAN_POINT('',(6.67,-3.2,2.));
#5273=CARTESIAN_POINT('',(6.67,-3.2,-0.1));
#5274=CARTESIAN_POINT('Origin',(7.,-3.2,2.));
#5275=CARTESIAN_POINT('Origin',(-7.,3.2,-0.1));
#5276=CARTESIAN_POINT('',(-7.33,3.2,0.));
#5277=CARTESIAN_POINT('Origin',(-7.,3.2,0.));
#5278=CARTESIAN_POINT('',(-7.33,3.2,2.));
#5279=CARTESIAN_POINT('',(-7.33,3.2,-0.1));
#5280=CARTESIAN_POINT('Origin',(-7.,3.2,2.));
#5281=CARTESIAN_POINT('Origin',(-7.,-3.2,-0.1));
#5282=CARTESIAN_POINT('',(-7.33,-3.2,0.));
#5283=CARTESIAN_POINT('Origin',(-7.,-3.2,0.));
#5284=CARTESIAN_POINT('',(-7.33,-3.2,2.));
#5285=CARTESIAN_POINT('',(-7.33,-3.2,-0.1));
#5286=CARTESIAN_POINT('Origin',(-7.,-3.2,2.));
#5287=CARTESIAN_POINT('Origin',(7.,3.2,-0.1));
#5288=CARTESIAN_POINT('',(6.67,3.2,0.));
#5289=CARTESIAN_POINT('Origin',(7.,3.2,0.));
#5290=CARTESIAN_POINT('',(6.67,3.2,2.));
#5291=CARTESIAN_POINT('',(6.67,3.2,-0.1));
#5292=CARTESIAN_POINT('Origin',(7.,3.2,2.));
#5293=CARTESIAN_POINT('Origin',(6.6,-1.5,1.));
#5294=CARTESIAN_POINT('',(6.6,-1.5,1.685));
#5295=CARTESIAN_POINT('Origin',(6.6,-1.5,1.));
#5296=CARTESIAN_POINT('',(8.,-1.5,1.685));
#5297=CARTESIAN_POINT('',(6.6,-1.5,1.685));
#5298=CARTESIAN_POINT('Origin',(8.,-1.5,1.));
#5299=CARTESIAN_POINT('Origin',(6.6,-1.5,1.));
#5300=CARTESIAN_POINT('',(6.6,-1.5,1.3));
#5301=CARTESIAN_POINT('Origin',(6.6,-1.5,1.));
#5302=CARTESIAN_POINT('Origin',(6.6,0.,1.));
#5303=CARTESIAN_POINT('',(6.6,-8.38883057415937E-17,1.685));
#5304=CARTESIAN_POINT('Origin',(6.6,0.,1.));
#5305=CARTESIAN_POINT('',(8.,8.38883057415937E-17,1.685));
#5306=CARTESIAN_POINT('',(6.6,-8.38883057415937E-17,1.685));
#5307=CARTESIAN_POINT('Origin',(8.,0.,1.));
#5308=CARTESIAN_POINT('Origin',(6.6,0.,1.));
#5309=CARTESIAN_POINT('',(6.6,-3.67394039744206E-17,1.3));
#5310=CARTESIAN_POINT('Origin',(6.6,0.,1.));
#5311=CARTESIAN_POINT('Origin',(6.6,1.5,1.));
#5312=CARTESIAN_POINT('',(6.6,1.5,1.685));
#5313=CARTESIAN_POINT('Origin',(6.6,1.5,1.));
#5314=CARTESIAN_POINT('',(8.,1.5,1.685));
#5315=CARTESIAN_POINT('',(6.6,1.5,1.685));
#5316=CARTESIAN_POINT('Origin',(8.,1.5,1.));
#5317=CARTESIAN_POINT('Origin',(6.6,1.5,1.));
#5318=CARTESIAN_POINT('',(6.6,1.5,1.3));
#5319=CARTESIAN_POINT('Origin',(6.6,1.5,1.));
#5320=CARTESIAN_POINT('Origin',(-8.1,-1.5,1.));
#5321=CARTESIAN_POINT('',(-8.,-1.5,1.685));
#5322=CARTESIAN_POINT('Origin',(-8.,-1.5,1.));
#5323=CARTESIAN_POINT('',(-6.6,-1.5,1.685));
#5324=CARTESIAN_POINT('',(-8.1,-1.5,1.685));
#5325=CARTESIAN_POINT('Origin',(-6.6,-1.5,1.));
#5326=CARTESIAN_POINT('Origin',(-6.6,-1.5,1.));
#5327=CARTESIAN_POINT('',(-6.6,-1.5,1.3));
#5328=CARTESIAN_POINT('Origin',(-6.6,-1.5,1.));
#5329=CARTESIAN_POINT('Origin',(-8.1,0.,1.));
#5330=CARTESIAN_POINT('',(-8.,-8.38883057415937E-17,1.685));
#5331=CARTESIAN_POINT('Origin',(-8.,0.,1.));
#5332=CARTESIAN_POINT('',(-6.6,-8.38883057415937E-17,1.685));
#5333=CARTESIAN_POINT('',(-8.1,-8.38883057415937E-17,1.685));
#5334=CARTESIAN_POINT('Origin',(-6.6,0.,1.));
#5335=CARTESIAN_POINT('Origin',(-6.6,0.,1.));
#5336=CARTESIAN_POINT('',(-6.6,3.67394039744206E-17,1.3));
#5337=CARTESIAN_POINT('Origin',(-6.6,0.,1.));
#5338=CARTESIAN_POINT('Origin',(-8.1,1.5,1.));
#5339=CARTESIAN_POINT('',(-8.,1.5,1.685));
#5340=CARTESIAN_POINT('Origin',(-8.,1.5,1.));
#5341=CARTESIAN_POINT('',(-6.6,1.5,1.685));
#5342=CARTESIAN_POINT('',(-8.1,1.5,1.685));
#5343=CARTESIAN_POINT('Origin',(-6.6,1.5,1.));
#5344=CARTESIAN_POINT('Origin',(-6.6,1.5,1.));
#5345=CARTESIAN_POINT('',(-6.6,1.5,1.3));
#5346=CARTESIAN_POINT('Origin',(-6.6,1.5,1.));
#5347=CARTESIAN_POINT('Origin',(-8.1,-1.5,1.));
#5348=CARTESIAN_POINT('',(-8.1,-1.5,1.3));
#5349=CARTESIAN_POINT('',(-8.1,-1.5,1.3));
#5350=CARTESIAN_POINT('',(-8.1,-1.5,1.3));
#5351=CARTESIAN_POINT('Origin',(-8.1,0.,1.));
#5352=CARTESIAN_POINT('',(-8.1,-3.67394039744206E-17,1.3));
#5353=CARTESIAN_POINT('',(-8.1,-3.67394039744206E-17,1.3));
#5354=CARTESIAN_POINT('',(-8.1,-3.67394039744206E-17,1.3));
#5355=CARTESIAN_POINT('Origin',(-8.1,1.5,1.));
#5356=CARTESIAN_POINT('',(-8.1,1.5,1.3));
#5357=CARTESIAN_POINT('',(-8.1,1.5,1.3));
#5358=CARTESIAN_POINT('',(-8.1,1.5,1.3));
#5359=CARTESIAN_POINT('Origin',(8.,4.,0.));
#5360=CARTESIAN_POINT('',(8.,4.,0.));
#5361=CARTESIAN_POINT('',(-8.,4.,0.));
#5362=CARTESIAN_POINT('',(8.,4.,0.));
#5363=CARTESIAN_POINT('',(-8.,4.,2.));
#5364=CARTESIAN_POINT('',(-8.,4.,0.));
#5365=CARTESIAN_POINT('',(8.,4.,2.));
#5366=CARTESIAN_POINT('',(8.,4.,2.));
#5367=CARTESIAN_POINT('',(8.,4.,0.));
#5368=CARTESIAN_POINT('Origin',(8.,-4.,0.));
#5369=CARTESIAN_POINT('',(8.,-4.,0.));
#5370=CARTESIAN_POINT('',(8.,-4.,0.));
#5371=CARTESIAN_POINT('',(8.,-4.,2.));
#5372=CARTESIAN_POINT('',(8.,-4.,2.));
#5373=CARTESIAN_POINT('',(8.,-4.,0.));
#5374=CARTESIAN_POINT('Origin',(-8.,-4.,0.));
#5375=CARTESIAN_POINT('',(-8.,-4.,0.));
#5376=CARTESIAN_POINT('',(-8.,-4.,0.));
#5377=CARTESIAN_POINT('',(-8.,-4.,2.));
#5378=CARTESIAN_POINT('',(-8.,-4.,2.));
#5379=CARTESIAN_POINT('',(-8.,-4.,0.));
#5380=CARTESIAN_POINT('Origin',(-8.,4.,0.));
#5381=CARTESIAN_POINT('',(-8.,4.,0.));
#5382=CARTESIAN_POINT('',(-8.,4.,2.));
#5383=CARTESIAN_POINT('Origin',(0.,0.,2.));
#5384=CARTESIAN_POINT('Origin',(0.,0.,0.));
#6083=UNCERTAINTY_MEASURE_WITH_UNIT(LENGTH_MEASURE(0.001),#6114,
'DISTANCE_ACCURACY_VALUE',
'Maximum model space distance between geometric entities at asserted c
onnectivities');
#6097=UNCERTAINTY_MEASURE_WITH_UNIT(LENGTH_MEASURE(0.001),#6114,
'DISTANCE_ACCURACY_VALUE',
'Maximum model space distance between geometric entities at asserted c
onnectivities');
#6099=(
GEOMETRIC_REPRESENTATION_CONTEXT(3)
GLOBAL_UNCERTAINTY_ASSIGNED_CONTEXT((#6083))
GLOBAL_UNIT_ASSIGNED_CONTEXT((#6114,#6116,#6117))
REPRESENTATION_CONTEXT('','3D')
);
#6113=(
GEOMETRIC_REPRESENTATION_CONTEXT(3)
GLOBAL_UNCERTAINTY_ASSIGNED_CONTEXT((#6097))
GLOBAL_UNIT_ASSIGNED_CONTEXT((#6114,#6116,#6117))
REPRESENTATION_CONTEXT('','3D')
);
#6114=(
LENGTH_UNIT()
NAMED_UNIT(*)
SI_UNIT(.CENTI.,.METRE.)
);
#6116=(
NAMED_UNIT(*)
PLANE_ANGLE_UNIT()
SI_UNIT($,.RADIAN.)
);
#6117=(
NAMED_UNIT(*)
SI_UNIT($,.STERADIAN.)
SOLID_ANGLE_UNIT()
);
#6119=SHAPE_DEFINITION_REPRESENTATION(#6134,#6168);
#6134=PRODUCT_DEFINITION_SHAPE('',$,#6184);
#6168=SHAPE_REPRESENTATION('',(#3505),#6099);
#6182=PRODUCT_DEFINITION_CONTEXT('part definition',#6229,'design');
#6184=PRODUCT_DEFINITION('Valve sub-base','Valve sub-base',#6199,
#6182);
#6199=PRODUCT_DEFINITION_FORMATION('',$,#6232);
#6229=APPLICATION_CONTEXT(
'Core Data for Automotive Mechanical Design Process');
#6230=PRODUCT_CONTEXT('part definition',#6229,'mechanical');
#6232=PRODUCT('Valve sub-base','Valve sub-base',
'Valve sub-base',(#6230));
#6288=COLOUR_RGB('Dark Blue',0.08,0.2,0.34);
#6289=FILL_AREA_STYLE_COLOUR('',#6288);
#6290=FILL_AREA_STYLE('',(#6289));
#6291=SURFACE_STYLE_FILL_AREA(#6290);
#6292=SURFACE_SIDE_STYLE('',(#6291));
#6293=SURFACE_STYLE_USAGE(.BOTH.,#6292);
#6294=PRESENTATION_STYLE_ASSIGNMENT((#6293));
ENDSEC;
END-ISO-10303-21;
